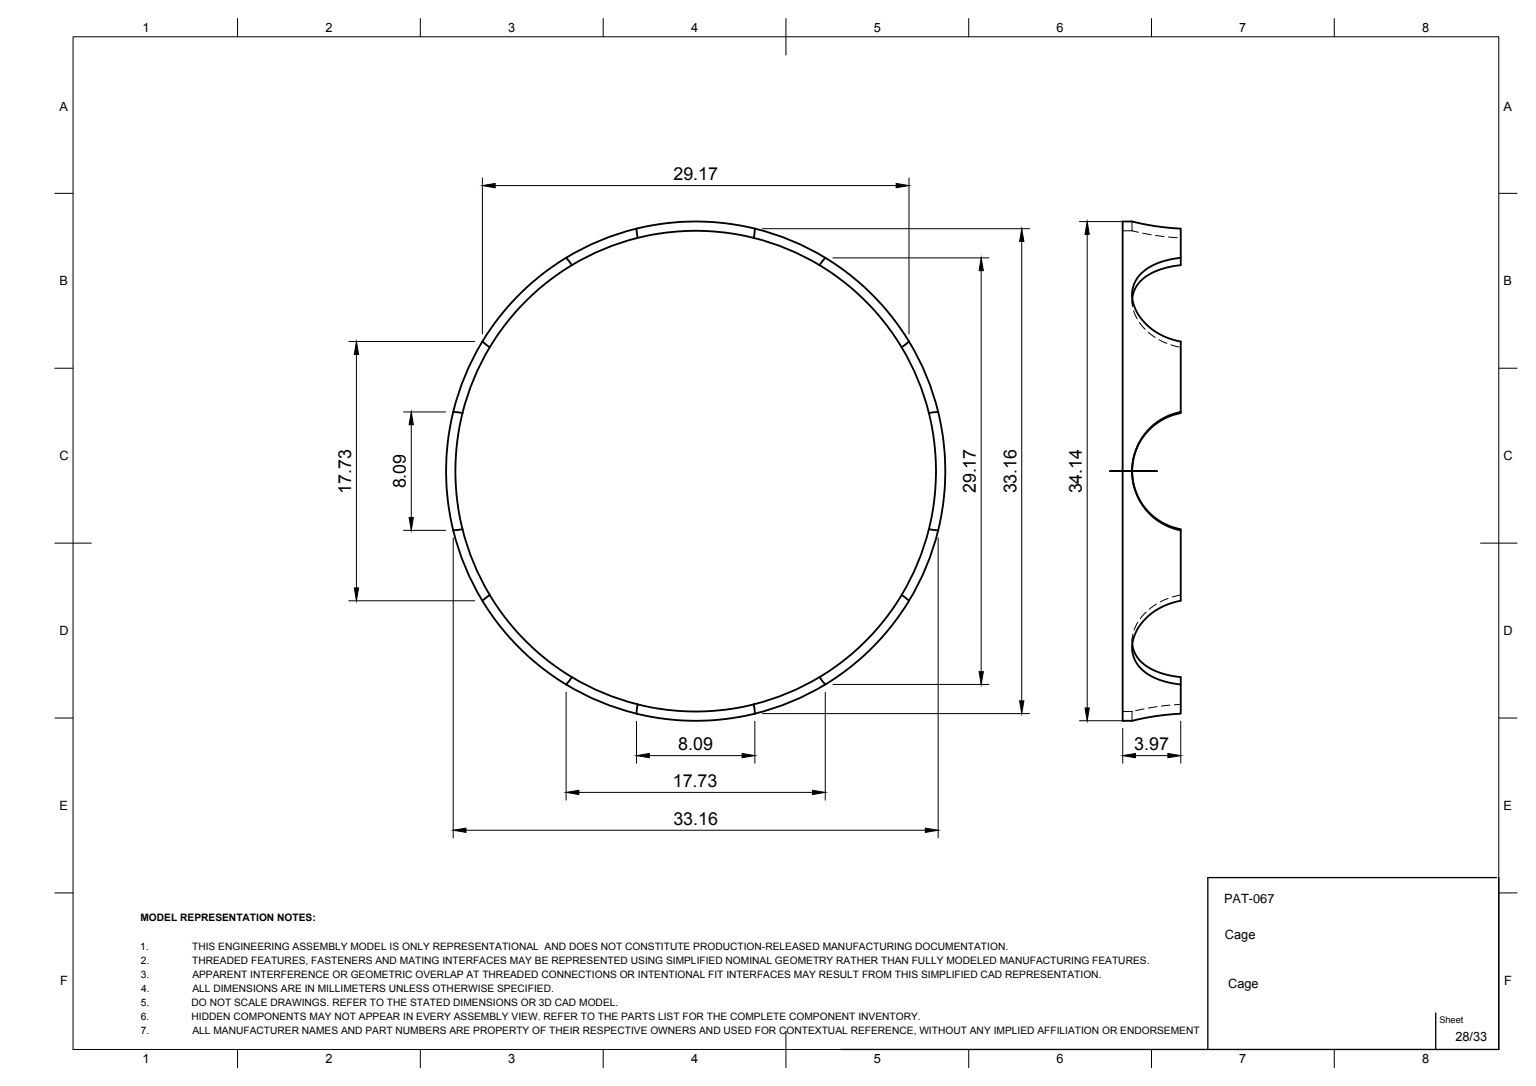
ISO-10303-21;
HEADER;
/* Generated by software containing ST-Developer
 * from STEP Tools, Inc. (www.steptools.com) 
 */

FILE_DESCRIPTION(
/* description */ ('Lifting hook block with sheave'),
/* implementation_level */ '2;1');

FILE_NAME(
/* name */ 'Cage.step',
/* time_stamp */ '2026-10-28T03:23:54-07:00',
/* author */ (''),
/* organization */ (''),
/* preprocessor_version */ 'ST-DEVELOPER v20.2',
/* originating_system */ 'Autodesk Translation Framework v15.17.0.0',
/* authorisation */ '');

FILE_SCHEMA (('AUTOMOTIVE_DESIGN { 1 0 10303 214 3 1 1 }'));
ENDSEC;

DATA;
#10=MECHANICAL_DESIGN_GEOMETRIC_PRESENTATION_REPRESENTATION('',(#381),#9391);
#11=B_SPLINE_CURVE_WITH_KNOTS('',3,(#8590,#8591,#8592,#8593,#8594,#8595,
#8596,#8597,#8598,#8599,#8600,#8601,#8602,#8603,#8604,#8605,#8606,#8607,
#8608,#8609,#8610,#8611),.UNSPECIFIED.,.F.,.F.,(4,2,2,2,2,2,2,2,2,2,4),
(0.0789094028588958,0.210573405340968,0.315860108011452,0.421146810681936,
0.522142632548711,0.623138454415485,0.72413427628226,0.825130098149035,
0.930416800819519,1.03570350349,1.16736750597208),.UNSPECIFIED.);
#12=B_SPLINE_CURVE_WITH_KNOTS('',3,(#8615,#8616,#8617,#8618,#8619,#8620,
#8621,#8622,#8623,#8624,#8625,#8626,#8627,#8628,#8629,#8630,#8631,#8632,
#8633,#8634,#8635,#8636),.UNSPECIFIED.,.F.,.F.,(4,2,2,2,2,2,2,2,2,2,4),
(0.0774793363974613,0.142088896491891,0.284177792983782,0.411119756996526,
0.514392970548519,0.617666184100513,0.720939397652506,0.8242126112045,0.951154575217244,
1.09324347170913,1.15785303180356),.UNSPECIFIED.);
#13=B_SPLINE_CURVE_WITH_KNOTS('',3,(#8642,#8643,#8644,#8645,#8646,#8647,
#8648,#8649,#8650,#8651,#8652,#8653,#8654,#8655,#8656,#8657,#8658,#8659,
#8660,#8661,#8662,#8663),.UNSPECIFIED.,.F.,.F.,(4,2,2,2,2,2,2,2,2,2,4),
(0.0774793363974613,0.142088896491891,0.284177792983782,0.411119756996525,
0.514392970548519,0.617666184100513,0.720939397652506,0.8242126112045,0.951154575217243,
1.09324347170913,1.15785303180356),.UNSPECIFIED.);
#14=B_SPLINE_CURVE_WITH_KNOTS('',3,(#8667,#8668,#8669,#8670,#8671,#8672,
#8673,#8674,#8675,#8676,#8677,#8678,#8679,#8680,#8681,#8682,#8683,#8684,
#8685,#8686,#8687,#8688),.UNSPECIFIED.,.F.,.F.,(4,2,2,2,2,2,2,2,2,2,4),
(0.0774793363974614,0.142088896491891,0.284177792983781,0.411119756996525,
0.514392970548519,0.617666184100512,0.720939397652506,0.824212611204499,
0.951154575217243,1.09324347170913,1.15785303180356),.UNSPECIFIED.);
#15=B_SPLINE_CURVE_WITH_KNOTS('',3,(#8692,#8693,#8694,#8695,#8696,#8697,
#8698,#8699,#8700,#8701,#8702,#8703),.UNSPECIFIED.,.F.,.F.,(4,2,2,2,2,4),
(0.0774793363974613,0.142088896491891,0.284177792983781,0.411119756996525,
0.514392970548519,0.617666184100512),.UNSPECIFIED.);
#16=B_SPLINE_CURVE_WITH_KNOTS('',3,(#8708,#8709,#8710,#8711,#8712,#8713,
#8714,#8715,#8716,#8717,#8718,#8719),.UNSPECIFIED.,.F.,.F.,(4,2,2,2,2,4),
(0.617666184100512,0.720939397652506,0.824212611204499,0.951154575217243,
1.09324347170913,1.15785303180356),.UNSPECIFIED.);
#17=B_SPLINE_CURVE_WITH_KNOTS('',3,(#8723,#8724,#8725,#8726,#8727,#8728,
#8729,#8730,#8731,#8732,#8733,#8734,#8735,#8736,#8737,#8738,#8739,#8740,
#8741,#8742,#8743,#8744),.UNSPECIFIED.,.F.,.F.,(4,2,2,2,2,2,2,2,2,2,4),
(0.0774793363974613,0.142088896491891,0.284177792983782,0.411119756996526,
0.514392970548519,0.617666184100513,0.720939397652507,0.8242126112045,0.951154575217245,
1.09324347170914,1.15785303180356),.UNSPECIFIED.);
#18=B_SPLINE_CURVE_WITH_KNOTS('',3,(#8748,#8749,#8750,#8751,#8752,#8753,
#8754,#8755,#8756,#8757,#8758,#8759,#8760,#8761,#8762,#8763,#8764,#8765,
#8766,#8767,#8768,#8769),.UNSPECIFIED.,.F.,.F.,(4,2,2,2,2,2,2,2,2,2,4),
(0.0774793363974613,0.142088896491891,0.284177792983782,0.411119756996526,
0.514392970548519,0.617666184100513,0.720939397652506,0.824212611204499,
0.951154575217243,1.09324347170913,1.15785303180356),.UNSPECIFIED.);
#19=B_SPLINE_CURVE_WITH_KNOTS('',3,(#8773,#8774,#8775,#8776,#8777,#8778,
#8779,#8780,#8781,#8782,#8783,#8784,#8785,#8786,#8787,#8788,#8789,#8790,
#8791,#8792,#8793,#8794),.UNSPECIFIED.,.F.,.F.,(4,2,2,2,2,2,2,2,2,2,4),
(0.0774793363974613,0.142088896491891,0.284177792983782,0.411119756996526,
0.514392970548519,0.617666184100513,0.720939397652506,0.8242126112045,0.951154575217244,
1.09324347170913,1.15785303180356),.UNSPECIFIED.);
#20=B_SPLINE_CURVE_WITH_KNOTS('',3,(#8798,#8799,#8800,#8801,#8802,#8803,
#8804,#8805,#8806,#8807,#8808,#8809,#8810,#8811,#8812,#8813,#8814,#8815,
#8816,#8817,#8818,#8819),.UNSPECIFIED.,.F.,.F.,(4,2,2,2,2,2,2,2,2,2,4),
(0.0774793363974613,0.142088896491891,0.284177792983782,0.411119756996526,
0.514392970548519,0.617666184100513,0.720939397652506,0.8242126112045,0.951154575217243,
1.09324347170913,1.15785303180356),.UNSPECIFIED.);
#21=B_SPLINE_CURVE_WITH_KNOTS('',3,(#8827,#8828,#8829,#8830,#8831,#8832,
#8833,#8834,#8835,#8836,#8837,#8838,#8839,#8840,#8841,#8842,#8843,#8844,
#8845,#8846,#8847,#8848),.UNSPECIFIED.,.F.,.F.,(4,2,2,2,2,2,2,2,2,2,4),
(0.0789094028588958,0.210573405340968,0.315860108011452,0.421146810681936,
0.522142632548711,0.623138454415485,0.72413427628226,0.825130098149035,
0.930416800819519,1.03570350349,1.16736750597208),.UNSPECIFIED.);
#22=B_SPLINE_CURVE_WITH_KNOTS('',3,(#8856,#8857,#8858,#8859,#8860,#8861,
#8862,#8863,#8864,#8865,#8866,#8867,#8868,#8869,#8870,#8871,#8872,#8873,
#8874,#8875,#8876,#8877),.UNSPECIFIED.,.F.,.F.,(4,2,2,2,2,2,2,2,2,2,4),
(0.0789094028588958,0.210573405340969,0.315860108011453,0.421146810681937,
0.522142632548712,0.623138454415486,0.724134276282261,0.825130098149035,
0.930416800819519,1.03570350349,1.16736750597208),.UNSPECIFIED.);
#23=B_SPLINE_CURVE_WITH_KNOTS('',3,(#8886,#8887,#8888,#8889,#8890,#8891,
#8892,#8893,#8894,#8895,#8896,#8897),.UNSPECIFIED.,.F.,.F.,(4,2,2,2,2,4),
(0.0789094028588958,0.210573405340968,0.315860108011452,0.421146810681937,
0.522142632548711,0.623138454415486),.UNSPECIFIED.);
#24=B_SPLINE_CURVE_WITH_KNOTS('',3,(#8899,#8900,#8901,#8902,#8903,#8904,
#8905,#8906,#8907,#8908,#8909,#8910),.UNSPECIFIED.,.F.,.F.,(4,2,2,2,2,4),
(0.623138454415486,0.72413427628226,0.825130098149035,0.930416800819519,
1.03570350349,1.16736750597208),.UNSPECIFIED.);
#25=B_SPLINE_CURVE_WITH_KNOTS('',3,(#8917,#8918,#8919,#8920,#8921,#8922,
#8923,#8924,#8925,#8926,#8927,#8928,#8929,#8930,#8931,#8932,#8933,#8934,
#8935,#8936,#8937,#8938),.UNSPECIFIED.,.F.,.F.,(4,2,2,2,2,2,2,2,2,2,4),
(0.0789094028588958,0.210573405340968,0.315860108011452,0.421146810681936,
0.522142632548711,0.623138454415486,0.72413427628226,0.825130098149035,
0.930416800819519,1.03570350349,1.16736750597208),.UNSPECIFIED.);
#26=B_SPLINE_CURVE_WITH_KNOTS('',3,(#8946,#8947,#8948,#8949,#8950,#8951,
#8952,#8953,#8954,#8955,#8956,#8957,#8958,#8959,#8960,#8961,#8962,#8963,
#8964,#8965,#8966,#8967),.UNSPECIFIED.,.F.,.F.,(4,2,2,2,2,2,2,2,2,2,4),
(0.0789094028588957,0.210573405340968,0.315860108011452,0.421146810681936,
0.522142632548711,0.623138454415485,0.72413427628226,0.825130098149035,
0.930416800819519,1.03570350349,1.16736750597207),.UNSPECIFIED.);
#27=B_SPLINE_CURVE_WITH_KNOTS('',3,(#8975,#8976,#8977,#8978,#8979,#8980,
#8981,#8982,#8983,#8984,#8985,#8986,#8987,#8988,#8989,#8990,#8991,#8992,
#8993,#8994,#8995,#8996),.UNSPECIFIED.,.F.,.F.,(4,2,2,2,2,2,2,2,2,2,4),
(0.0789094028588958,0.210573405340968,0.315860108011452,0.421146810681936,
0.522142632548711,0.623138454415486,0.72413427628226,0.825130098149035,
0.930416800819519,1.03570350349,1.16736750597208),.UNSPECIFIED.);
#28=B_SPLINE_CURVE_WITH_KNOTS('',3,(#9005,#9006,#9007,#9008,#9009,#9010,
#9011,#9012,#9013,#9014,#9015,#9016,#9017,#9018,#9019,#9020,#9021,#9022,
#9023,#9024,#9025,#9026),.UNSPECIFIED.,.F.,.F.,(4,2,2,2,2,2,2,2,2,2,4),
(0.0789094028588958,0.210573405340968,0.315860108011452,0.421146810681936,
0.522142632548711,0.623138454415485,0.72413427628226,0.825130098149035,
0.930416800819519,1.03570350349,1.16736750597208),.UNSPECIFIED.);
#37=SPHERICAL_SURFACE('',#5741,0.412776);
#38=SPHERICAL_SURFACE('',#5757,0.412776);
#39=SPHERICAL_SURFACE('',#5762,0.412776);
#40=SPHERICAL_SURFACE('',#5767,0.412776);
#41=SPHERICAL_SURFACE('',#5772,0.412776);
#42=SPHERICAL_SURFACE('',#5777,0.412776);
#43=SPHERICAL_SURFACE('',#5782,0.412776);
#44=SPHERICAL_SURFACE('',#5790,0.412776);
#314=SHAPE_REPRESENTATION_RELATIONSHIP('SRR','None',#9547,#344);
#344=ADVANCED_BREP_SHAPE_REPRESENTATION('',(#417),#9382);
#381=STYLED_ITEM('',(#9759),#417);
#417=MANIFOLD_SOLID_BREP('Continuous crown cage',#4919);
#636=LINE('',#8705,#924);
#637=LINE('',#9001,#925);
#924=VECTOR('',#7119,1.706752);
#925=VECTOR('',#7196,1.643248);
#1087=CYLINDRICAL_SURFACE('',#5744,1.706752);
#1088=CYLINDRICAL_SURFACE('',#5784,1.643248);
#1206=FACE_BOUND('',#1839,.T.);
#1433=FACE_OUTER_BOUND('',#1821,.T.);
#1434=FACE_OUTER_BOUND('',#1822,.T.);
#1435=FACE_OUTER_BOUND('',#1823,.T.);
#1436=FACE_OUTER_BOUND('',#1824,.T.);
#1437=FACE_OUTER_BOUND('',#1825,.T.);
#1438=FACE_OUTER_BOUND('',#1826,.T.);
#1439=FACE_OUTER_BOUND('',#1827,.T.);
#1440=FACE_OUTER_BOUND('',#1828,.T.);
#1441=FACE_OUTER_BOUND('',#1829,.T.);
#1442=FACE_OUTER_BOUND('',#1830,.T.);
#1443=FACE_OUTER_BOUND('',#1831,.T.);
#1444=FACE_OUTER_BOUND('',#1832,.T.);
#1445=FACE_OUTER_BOUND('',#1833,.T.);
#1446=FACE_OUTER_BOUND('',#1834,.T.);
#1447=FACE_OUTER_BOUND('',#1835,.T.);
#1448=FACE_OUTER_BOUND('',#1836,.T.);
#1449=FACE_OUTER_BOUND('',#1837,.T.);
#1450=FACE_OUTER_BOUND('',#1838,.T.);
#1451=FACE_OUTER_BOUND('',#1840,.T.);
#1821=EDGE_LOOP('',(#4114,#4115,#4116,#4117));
#1822=EDGE_LOOP('',(#4118,#4119,#4120,#4121,#4122,#4123,#4124,#4125,#4126,
#4127,#4128,#4129,#4130,#4131,#4132,#4133,#4134,#4135,#4136,#4137));
#1823=EDGE_LOOP('',(#4138,#4139,#4140,#4141));
#1824=EDGE_LOOP('',(#4142,#4143,#4144,#4145));
#1825=EDGE_LOOP('',(#4146,#4147,#4148,#4149));
#1826=EDGE_LOOP('',(#4150,#4151,#4152,#4153));
#1827=EDGE_LOOP('',(#4154,#4155,#4156,#4157));
#1828=EDGE_LOOP('',(#4158,#4159,#4160,#4161,#4162,#4163));
#1829=EDGE_LOOP('',(#4164,#4165,#4166,#4167));
#1830=EDGE_LOOP('',(#4168,#4169,#4170,#4171));
#1831=EDGE_LOOP('',(#4172,#4173,#4174,#4175));
#1832=EDGE_LOOP('',(#4176,#4177,#4178,#4179));
#1833=EDGE_LOOP('',(#4180,#4181,#4182,#4183));
#1834=EDGE_LOOP('',(#4184,#4185,#4186,#4187));
#1835=EDGE_LOOP('',(#4188,#4189,#4190,#4191,#4192,#4193,#4194,#4195,#4196,
#4197,#4198,#4199,#4200,#4201,#4202,#4203,#4204,#4205,#4206,#4207));
#1836=EDGE_LOOP('',(#4208,#4209,#4210,#4211));
#1837=EDGE_LOOP('',(#4212,#4213,#4214,#4215));
#1838=EDGE_LOOP('',(#4216));
#1839=EDGE_LOOP('',(#4217));
#1840=EDGE_LOOP('',(#4218,#4219,#4220,#4221));
#2133=CIRCLE('',#5742,0.405071403305639);
#2134=CIRCLE('',#5743,0.405071403305639);
#2135=CIRCLE('',#5745,1.706752);
#2136=CIRCLE('',#5746,1.706752);
#2137=CIRCLE('',#5747,1.706752);
#2138=CIRCLE('',#5748,1.706752);
#2139=CIRCLE('',#5749,1.706752);
#2140=CIRCLE('',#5750,1.706752);
#2141=CIRCLE('',#5751,1.706752);
#2142=CIRCLE('',#5752,1.706752);
#2143=CIRCLE('',#5753,1.706752);
#2144=CIRCLE('',#5755,1.643248);
#2145=CIRCLE('',#5756,0.405071403305639);
#2146=CIRCLE('',#5758,0.405071403305639);
#2147=CIRCLE('',#5760,1.643248);
#2148=CIRCLE('',#5761,0.405071403305639);
#2149=CIRCLE('',#5763,0.405071403305639);
#2150=CIRCLE('',#5765,1.643248);
#2151=CIRCLE('',#5766,0.405071403305639);
#2152=CIRCLE('',#5768,0.405071403305639);
#2153=CIRCLE('',#5770,1.643248);
#2154=CIRCLE('',#5771,0.405071403305639);
#2155=CIRCLE('',#5773,0.405071403305639);
#2156=CIRCLE('',#5775,1.643248);
#2157=CIRCLE('',#5776,0.405071403305639);
#2158=CIRCLE('',#5778,0.405071403305639);
#2159=CIRCLE('',#5780,1.643248);
#2160=CIRCLE('',#5781,0.405071403305639);
#2161=CIRCLE('',#5783,0.405071403305639);
#2162=CIRCLE('',#5785,1.643248);
#2163=CIRCLE('',#5786,1.643248);
#2164=CIRCLE('',#5787,1.643248);
#2165=CIRCLE('',#5789,0.405071403305639);
#2166=CIRCLE('',#5791,0.405071403305639);
#2508=VERTEX_POINT('',#8588);
#2509=VERTEX_POINT('',#8589);
#2510=VERTEX_POINT('',#8612);
#2511=VERTEX_POINT('',#8614);
#2512=VERTEX_POINT('',#8639);
#2513=VERTEX_POINT('',#8641);
#2514=VERTEX_POINT('',#8664);
#2515=VERTEX_POINT('',#8666);
#2516=VERTEX_POINT('',#8689);
#2517=VERTEX_POINT('',#8691);
#2518=VERTEX_POINT('',#8704);
#2519=VERTEX_POINT('',#8707);
#2520=VERTEX_POINT('',#8720);
#2521=VERTEX_POINT('',#8722);
#2522=VERTEX_POINT('',#8745);
#2523=VERTEX_POINT('',#8747);
#2524=VERTEX_POINT('',#8770);
#2525=VERTEX_POINT('',#8772);
#2526=VERTEX_POINT('',#8795);
#2527=VERTEX_POINT('',#8797);
#2528=VERTEX_POINT('',#8822);
#2529=VERTEX_POINT('',#8826);
#2530=VERTEX_POINT('',#8851);
#2531=VERTEX_POINT('',#8855);
#2532=VERTEX_POINT('',#8880);
#2533=VERTEX_POINT('',#8884);
#2534=VERTEX_POINT('',#8885);
#2535=VERTEX_POINT('',#8912);
#2536=VERTEX_POINT('',#8916);
#2537=VERTEX_POINT('',#8941);
#2538=VERTEX_POINT('',#8945);
#2539=VERTEX_POINT('',#8970);
#2540=VERTEX_POINT('',#8974);
#2541=VERTEX_POINT('',#8999);
#2542=VERTEX_POINT('',#9002);
#2543=VERTEX_POINT('',#9004);
#3061=EDGE_CURVE('',#2508,#2509,#11,.T.);
#3062=EDGE_CURVE('',#2510,#2508,#2133,.T.);
#3063=EDGE_CURVE('',#2511,#2510,#12,.T.);
#3064=EDGE_CURVE('',#2509,#2511,#2134,.T.);
#3065=EDGE_CURVE('',#2512,#2510,#2135,.T.);
#3066=EDGE_CURVE('',#2512,#2513,#13,.T.);
#3067=EDGE_CURVE('',#2514,#2513,#2136,.T.);
#3068=EDGE_CURVE('',#2514,#2515,#14,.T.);
#3069=EDGE_CURVE('',#2516,#2515,#2137,.T.);
#3070=EDGE_CURVE('',#2516,#2517,#15,.T.);
#3071=EDGE_CURVE('',#2517,#2518,#636,.T.);
#3072=EDGE_CURVE('',#2518,#2518,#2138,.T.);
#3073=EDGE_CURVE('',#2517,#2519,#16,.T.);
#3074=EDGE_CURVE('',#2520,#2519,#2139,.T.);
#3075=EDGE_CURVE('',#2520,#2521,#17,.T.);
#3076=EDGE_CURVE('',#2522,#2521,#2140,.T.);
#3077=EDGE_CURVE('',#2522,#2523,#18,.T.);
#3078=EDGE_CURVE('',#2524,#2523,#2141,.T.);
#3079=EDGE_CURVE('',#2524,#2525,#19,.T.);
#3080=EDGE_CURVE('',#2526,#2525,#2142,.T.);
#3081=EDGE_CURVE('',#2526,#2527,#20,.T.);
#3082=EDGE_CURVE('',#2511,#2527,#2143,.T.);
#3083=EDGE_CURVE('',#2508,#2528,#2144,.T.);
#3084=EDGE_CURVE('',#2528,#2512,#2145,.T.);
#3085=EDGE_CURVE('',#2529,#2528,#21,.T.);
#3086=EDGE_CURVE('',#2513,#2529,#2146,.T.);
#3087=EDGE_CURVE('',#2529,#2530,#2147,.T.);
#3088=EDGE_CURVE('',#2530,#2514,#2148,.T.);
#3089=EDGE_CURVE('',#2531,#2530,#22,.T.);
#3090=EDGE_CURVE('',#2515,#2531,#2149,.T.);
#3091=EDGE_CURVE('',#2531,#2532,#2150,.T.);
#3092=EDGE_CURVE('',#2532,#2516,#2151,.T.);
#3093=EDGE_CURVE('',#2533,#2534,#23,.T.);
#3094=EDGE_CURVE('',#2519,#2533,#2152,.T.);
#3095=EDGE_CURVE('',#2534,#2532,#24,.T.);
#3096=EDGE_CURVE('',#2533,#2535,#2153,.T.);
#3097=EDGE_CURVE('',#2535,#2520,#2154,.T.);
#3098=EDGE_CURVE('',#2536,#2535,#25,.T.);
#3099=EDGE_CURVE('',#2521,#2536,#2155,.T.);
#3100=EDGE_CURVE('',#2536,#2537,#2156,.T.);
#3101=EDGE_CURVE('',#2537,#2522,#2157,.T.);
#3102=EDGE_CURVE('',#2538,#2537,#26,.T.);
#3103=EDGE_CURVE('',#2523,#2538,#2158,.T.);
#3104=EDGE_CURVE('',#2538,#2539,#2159,.T.);
#3105=EDGE_CURVE('',#2539,#2524,#2160,.T.);
#3106=EDGE_CURVE('',#2540,#2539,#27,.T.);
#3107=EDGE_CURVE('',#2525,#2540,#2161,.T.);
#3108=EDGE_CURVE('',#2541,#2541,#2162,.T.);
#3109=EDGE_CURVE('',#2541,#2534,#637,.T.);
#3110=EDGE_CURVE('',#2542,#2509,#2163,.T.);
#3111=EDGE_CURVE('',#2542,#2543,#28,.T.);
#3112=EDGE_CURVE('',#2540,#2543,#2164,.T.);
#3113=EDGE_CURVE('',#2527,#2542,#2165,.T.);
#3114=EDGE_CURVE('',#2543,#2526,#2166,.T.);
#4114=ORIENTED_EDGE('',*,*,#3061,.F.);
#4115=ORIENTED_EDGE('',*,*,#3062,.F.);
#4116=ORIENTED_EDGE('',*,*,#3063,.F.);
#4117=ORIENTED_EDGE('',*,*,#3064,.F.);
#4118=ORIENTED_EDGE('',*,*,#3063,.T.);
#4119=ORIENTED_EDGE('',*,*,#3065,.F.);
#4120=ORIENTED_EDGE('',*,*,#3066,.T.);
#4121=ORIENTED_EDGE('',*,*,#3067,.F.);
#4122=ORIENTED_EDGE('',*,*,#3068,.T.);
#4123=ORIENTED_EDGE('',*,*,#3069,.F.);
#4124=ORIENTED_EDGE('',*,*,#3070,.T.);
#4125=ORIENTED_EDGE('',*,*,#3071,.T.);
#4126=ORIENTED_EDGE('',*,*,#3072,.F.);
#4127=ORIENTED_EDGE('',*,*,#3071,.F.);
#4128=ORIENTED_EDGE('',*,*,#3073,.T.);
#4129=ORIENTED_EDGE('',*,*,#3074,.F.);
#4130=ORIENTED_EDGE('',*,*,#3075,.T.);
#4131=ORIENTED_EDGE('',*,*,#3076,.F.);
#4132=ORIENTED_EDGE('',*,*,#3077,.T.);
#4133=ORIENTED_EDGE('',*,*,#3078,.F.);
#4134=ORIENTED_EDGE('',*,*,#3079,.T.);
#4135=ORIENTED_EDGE('',*,*,#3080,.F.);
#4136=ORIENTED_EDGE('',*,*,#3081,.T.);
#4137=ORIENTED_EDGE('',*,*,#3082,.F.);
#4138=ORIENTED_EDGE('',*,*,#3062,.T.);
#4139=ORIENTED_EDGE('',*,*,#3083,.T.);
#4140=ORIENTED_EDGE('',*,*,#3084,.T.);
#4141=ORIENTED_EDGE('',*,*,#3065,.T.);
#4142=ORIENTED_EDGE('',*,*,#3085,.F.);
#4143=ORIENTED_EDGE('',*,*,#3086,.F.);
#4144=ORIENTED_EDGE('',*,*,#3066,.F.);
#4145=ORIENTED_EDGE('',*,*,#3084,.F.);
#4146=ORIENTED_EDGE('',*,*,#3086,.T.);
#4147=ORIENTED_EDGE('',*,*,#3087,.T.);
#4148=ORIENTED_EDGE('',*,*,#3088,.T.);
#4149=ORIENTED_EDGE('',*,*,#3067,.T.);
#4150=ORIENTED_EDGE('',*,*,#3089,.F.);
#4151=ORIENTED_EDGE('',*,*,#3090,.F.);
#4152=ORIENTED_EDGE('',*,*,#3068,.F.);
#4153=ORIENTED_EDGE('',*,*,#3088,.F.);
#4154=ORIENTED_EDGE('',*,*,#3090,.T.);
#4155=ORIENTED_EDGE('',*,*,#3091,.T.);
#4156=ORIENTED_EDGE('',*,*,#3092,.T.);
#4157=ORIENTED_EDGE('',*,*,#3069,.T.);
#4158=ORIENTED_EDGE('',*,*,#3093,.F.);
#4159=ORIENTED_EDGE('',*,*,#3094,.F.);
#4160=ORIENTED_EDGE('',*,*,#3073,.F.);
#4161=ORIENTED_EDGE('',*,*,#3070,.F.);
#4162=ORIENTED_EDGE('',*,*,#3092,.F.);
#4163=ORIENTED_EDGE('',*,*,#3095,.F.);
#4164=ORIENTED_EDGE('',*,*,#3094,.T.);
#4165=ORIENTED_EDGE('',*,*,#3096,.T.);
#4166=ORIENTED_EDGE('',*,*,#3097,.T.);
#4167=ORIENTED_EDGE('',*,*,#3074,.T.);
#4168=ORIENTED_EDGE('',*,*,#3098,.F.);
#4169=ORIENTED_EDGE('',*,*,#3099,.F.);
#4170=ORIENTED_EDGE('',*,*,#3075,.F.);
#4171=ORIENTED_EDGE('',*,*,#3097,.F.);
#4172=ORIENTED_EDGE('',*,*,#3099,.T.);
#4173=ORIENTED_EDGE('',*,*,#3100,.T.);
#4174=ORIENTED_EDGE('',*,*,#3101,.T.);
#4175=ORIENTED_EDGE('',*,*,#3076,.T.);
#4176=ORIENTED_EDGE('',*,*,#3102,.F.);
#4177=ORIENTED_EDGE('',*,*,#3103,.F.);
#4178=ORIENTED_EDGE('',*,*,#3077,.F.);
#4179=ORIENTED_EDGE('',*,*,#3101,.F.);
#4180=ORIENTED_EDGE('',*,*,#3103,.T.);
#4181=ORIENTED_EDGE('',*,*,#3104,.T.);
#4182=ORIENTED_EDGE('',*,*,#3105,.T.);
#4183=ORIENTED_EDGE('',*,*,#3078,.T.);
#4184=ORIENTED_EDGE('',*,*,#3079,.F.);
#4185=ORIENTED_EDGE('',*,*,#3105,.F.);
#4186=ORIENTED_EDGE('',*,*,#3106,.F.);
#4187=ORIENTED_EDGE('',*,*,#3107,.F.);
#4188=ORIENTED_EDGE('',*,*,#3108,.F.);
#4189=ORIENTED_EDGE('',*,*,#3109,.T.);
#4190=ORIENTED_EDGE('',*,*,#3095,.T.);
#4191=ORIENTED_EDGE('',*,*,#3091,.F.);
#4192=ORIENTED_EDGE('',*,*,#3089,.T.);
#4193=ORIENTED_EDGE('',*,*,#3087,.F.);
#4194=ORIENTED_EDGE('',*,*,#3085,.T.);
#4195=ORIENTED_EDGE('',*,*,#3083,.F.);
#4196=ORIENTED_EDGE('',*,*,#3061,.T.);
#4197=ORIENTED_EDGE('',*,*,#3110,.F.);
#4198=ORIENTED_EDGE('',*,*,#3111,.T.);
#4199=ORIENTED_EDGE('',*,*,#3112,.F.);
#4200=ORIENTED_EDGE('',*,*,#3106,.T.);
#4201=ORIENTED_EDGE('',*,*,#3104,.F.);
#4202=ORIENTED_EDGE('',*,*,#3102,.T.);
#4203=ORIENTED_EDGE('',*,*,#3100,.F.);
#4204=ORIENTED_EDGE('',*,*,#3098,.T.);
#4205=ORIENTED_EDGE('',*,*,#3096,.F.);
#4206=ORIENTED_EDGE('',*,*,#3093,.T.);
#4207=ORIENTED_EDGE('',*,*,#3109,.F.);
#4208=ORIENTED_EDGE('',*,*,#3064,.T.);
#4209=ORIENTED_EDGE('',*,*,#3082,.T.);
#4210=ORIENTED_EDGE('',*,*,#3113,.T.);
#4211=ORIENTED_EDGE('',*,*,#3110,.T.);
#4212=ORIENTED_EDGE('',*,*,#3081,.F.);
#4213=ORIENTED_EDGE('',*,*,#3114,.F.);
#4214=ORIENTED_EDGE('',*,*,#3111,.F.);
#4215=ORIENTED_EDGE('',*,*,#3113,.F.);
#4216=ORIENTED_EDGE('',*,*,#3072,.T.);
#4217=ORIENTED_EDGE('',*,*,#3108,.T.);
#4218=ORIENTED_EDGE('',*,*,#3107,.T.);
#4219=ORIENTED_EDGE('',*,*,#3112,.T.);
#4220=ORIENTED_EDGE('',*,*,#3114,.T.);
#4221=ORIENTED_EDGE('',*,*,#3080,.T.);
#4551=PLANE('',#5754);
#4552=PLANE('',#5759);
#4553=PLANE('',#5764);
#4554=PLANE('',#5769);
#4555=PLANE('',#5774);
#4556=PLANE('',#5779);
#4557=PLANE('',#5788);
#4558=PLANE('',#5792);
#4559=PLANE('',#5793);
#4809=ADVANCED_FACE('',(#1433),#37,.F.);
#4810=ADVANCED_FACE('',(#1434),#1087,.T.);
#4811=ADVANCED_FACE('',(#1435),#4551,.T.);
#4812=ADVANCED_FACE('',(#1436),#38,.F.);
#4813=ADVANCED_FACE('',(#1437),#4552,.T.);
#4814=ADVANCED_FACE('',(#1438),#39,.F.);
#4815=ADVANCED_FACE('',(#1439),#4553,.T.);
#4816=ADVANCED_FACE('',(#1440),#40,.F.);
#4817=ADVANCED_FACE('',(#1441),#4554,.T.);
#4818=ADVANCED_FACE('',(#1442),#41,.F.);
#4819=ADVANCED_FACE('',(#1443),#4555,.T.);
#4820=ADVANCED_FACE('',(#1444),#42,.F.);
#4821=ADVANCED_FACE('',(#1445),#4556,.T.);
#4822=ADVANCED_FACE('',(#1446),#43,.F.);
#4823=ADVANCED_FACE('',(#1447),#1088,.F.);
#4824=ADVANCED_FACE('',(#1448),#4557,.T.);
#4825=ADVANCED_FACE('',(#1449),#44,.F.);
#4826=ADVANCED_FACE('',(#1450,#1206),#4558,.T.);
#4827=ADVANCED_FACE('',(#1451),#4559,.T.);
#4919=CLOSED_SHELL('',(#4809,#4810,#4811,#4812,#4813,#4814,#4815,#4816,
#4817,#4818,#4819,#4820,#4821,#4822,#4823,#4824,#4825,#4826,#4827));
#5740=AXIS2_PLACEMENT_3D('',#8586,#7103,#7104);
#5741=AXIS2_PLACEMENT_3D('',#8587,#7105,#7106);
#5742=AXIS2_PLACEMENT_3D('',#8613,#7107,#7108);
#5743=AXIS2_PLACEMENT_3D('',#8637,#7109,#7110);
#5744=AXIS2_PLACEMENT_3D('',#8638,#7111,#7112);
#5745=AXIS2_PLACEMENT_3D('',#8640,#7113,#7114);
#5746=AXIS2_PLACEMENT_3D('',#8665,#7115,#7116);
#5747=AXIS2_PLACEMENT_3D('',#8690,#7117,#7118);
#5748=AXIS2_PLACEMENT_3D('',#8706,#7120,#7121);
#5749=AXIS2_PLACEMENT_3D('',#8721,#7122,#7123);
#5750=AXIS2_PLACEMENT_3D('',#8746,#7124,#7125);
#5751=AXIS2_PLACEMENT_3D('',#8771,#7126,#7127);
#5752=AXIS2_PLACEMENT_3D('',#8796,#7128,#7129);
#5753=AXIS2_PLACEMENT_3D('',#8820,#7130,#7131);
#5754=AXIS2_PLACEMENT_3D('',#8821,#7132,#7133);
#5755=AXIS2_PLACEMENT_3D('',#8823,#7134,#7135);
#5756=AXIS2_PLACEMENT_3D('',#8824,#7136,#7137);
#5757=AXIS2_PLACEMENT_3D('',#8825,#7138,#7139);
#5758=AXIS2_PLACEMENT_3D('',#8849,#7140,#7141);
#5759=AXIS2_PLACEMENT_3D('',#8850,#7142,#7143);
#5760=AXIS2_PLACEMENT_3D('',#8852,#7144,#7145);
#5761=AXIS2_PLACEMENT_3D('',#8853,#7146,#7147);
#5762=AXIS2_PLACEMENT_3D('',#8854,#7148,#7149);
#5763=AXIS2_PLACEMENT_3D('',#8878,#7150,#7151);
#5764=AXIS2_PLACEMENT_3D('',#8879,#7152,#7153);
#5765=AXIS2_PLACEMENT_3D('',#8881,#7154,#7155);
#5766=AXIS2_PLACEMENT_3D('',#8882,#7156,#7157);
#5767=AXIS2_PLACEMENT_3D('',#8883,#7158,#7159);
#5768=AXIS2_PLACEMENT_3D('',#8898,#7160,#7161);
#5769=AXIS2_PLACEMENT_3D('',#8911,#7162,#7163);
#5770=AXIS2_PLACEMENT_3D('',#8913,#7164,#7165);
#5771=AXIS2_PLACEMENT_3D('',#8914,#7166,#7167);
#5772=AXIS2_PLACEMENT_3D('',#8915,#7168,#7169);
#5773=AXIS2_PLACEMENT_3D('',#8939,#7170,#7171);
#5774=AXIS2_PLACEMENT_3D('',#8940,#7172,#7173);
#5775=AXIS2_PLACEMENT_3D('',#8942,#7174,#7175);
#5776=AXIS2_PLACEMENT_3D('',#8943,#7176,#7177);
#5777=AXIS2_PLACEMENT_3D('',#8944,#7178,#7179);
#5778=AXIS2_PLACEMENT_3D('',#8968,#7180,#7181);
#5779=AXIS2_PLACEMENT_3D('',#8969,#7182,#7183);
#5780=AXIS2_PLACEMENT_3D('',#8971,#7184,#7185);
#5781=AXIS2_PLACEMENT_3D('',#8972,#7186,#7187);
#5782=AXIS2_PLACEMENT_3D('',#8973,#7188,#7189);
#5783=AXIS2_PLACEMENT_3D('',#8997,#7190,#7191);
#5784=AXIS2_PLACEMENT_3D('',#8998,#7192,#7193);
#5785=AXIS2_PLACEMENT_3D('',#9000,#7194,#7195);
#5786=AXIS2_PLACEMENT_3D('',#9003,#7197,#7198);
#5787=AXIS2_PLACEMENT_3D('',#9027,#7199,#7200);
#5788=AXIS2_PLACEMENT_3D('',#9028,#7201,#7202);
#5789=AXIS2_PLACEMENT_3D('',#9029,#7203,#7204);
#5790=AXIS2_PLACEMENT_3D('',#9030,#7205,#7206);
#5791=AXIS2_PLACEMENT_3D('',#9031,#7207,#7208);
#5792=AXIS2_PLACEMENT_3D('',#9032,#7209,#7210);
#5793=AXIS2_PLACEMENT_3D('',#9033,#7211,#7212);
#7103=DIRECTION('axis',(0.,0.,1.));
#7104=DIRECTION('refdir',(1.,0.,0.));
#7105=DIRECTION('center_axis',(0.,0.,1.));
#7106=DIRECTION('ref_axis',(1.,0.,0.));
#7107=DIRECTION('center_axis',(0.,-1.,0.));
#7108=DIRECTION('ref_axis',(0.,0.,-1.));
#7109=DIRECTION('center_axis',(0.,-1.,0.));
#7110=DIRECTION('ref_axis',(0.,0.,-1.));
#7111=DIRECTION('center_axis',(0.,1.,0.));
#7112=DIRECTION('ref_axis',(1.,0.,0.));
#7113=DIRECTION('center_axis',(0.,1.,0.));
#7114=DIRECTION('ref_axis',(1.,0.,0.));
#7115=DIRECTION('center_axis',(0.,1.,0.));
#7116=DIRECTION('ref_axis',(1.,0.,0.));
#7117=DIRECTION('center_axis',(0.,1.,0.));
#7118=DIRECTION('ref_axis',(1.,0.,0.));
#7119=DIRECTION('',(0.,-1.,0.));
#7120=DIRECTION('center_axis',(0.,-1.,0.));
#7121=DIRECTION('ref_axis',(1.,0.,0.));
#7122=DIRECTION('center_axis',(0.,1.,0.));
#7123=DIRECTION('ref_axis',(1.,0.,0.));
#7124=DIRECTION('center_axis',(0.,1.,0.));
#7125=DIRECTION('ref_axis',(1.,0.,0.));
#7126=DIRECTION('center_axis',(0.,1.,0.));
#7127=DIRECTION('ref_axis',(1.,0.,0.));
#7128=DIRECTION('center_axis',(0.,1.,0.));
#7129=DIRECTION('ref_axis',(1.,0.,0.));
#7130=DIRECTION('center_axis',(0.,1.,0.));
#7131=DIRECTION('ref_axis',(1.,0.,0.));
#7132=DIRECTION('center_axis',(0.,1.,0.));
#7133=DIRECTION('ref_axis',(1.,0.,0.));
#7134=DIRECTION('center_axis',(0.,-1.,0.));
#7135=DIRECTION('ref_axis',(1.,0.,0.));
#7136=DIRECTION('center_axis',(0.,-1.,0.));
#7137=DIRECTION('ref_axis',(0.,0.,-1.));
#7138=DIRECTION('center_axis',(6.12323399573677E-17,0.,1.));
#7139=DIRECTION('ref_axis',(1.,0.,0.));
#7140=DIRECTION('center_axis',(0.,-1.,0.));
#7141=DIRECTION('ref_axis',(0.,0.,-1.));
#7142=DIRECTION('center_axis',(0.,1.,0.));
#7143=DIRECTION('ref_axis',(1.,0.,0.));
#7144=DIRECTION('center_axis',(0.,-1.,0.));
#7145=DIRECTION('ref_axis',(1.,0.,0.));
#7146=DIRECTION('center_axis',(0.,-1.,0.));
#7147=DIRECTION('ref_axis',(0.,0.,-1.));
#7148=DIRECTION('center_axis',(0.,0.,1.));
#7149=DIRECTION('ref_axis',(1.,0.,0.));
#7150=DIRECTION('center_axis',(0.,-1.,0.));
#7151=DIRECTION('ref_axis',(0.,0.,-1.));
#7152=DIRECTION('center_axis',(0.,1.,0.));
#7153=DIRECTION('ref_axis',(1.,0.,0.));
#7154=DIRECTION('center_axis',(0.,-1.,0.));
#7155=DIRECTION('ref_axis',(1.,0.,0.));
#7156=DIRECTION('center_axis',(0.,-1.,0.));
#7157=DIRECTION('ref_axis',(0.,0.,-1.));
#7158=DIRECTION('center_axis',(0.,0.,1.));
#7159=DIRECTION('ref_axis',(1.,0.,0.));
#7160=DIRECTION('center_axis',(0.,-1.,0.));
#7161=DIRECTION('ref_axis',(0.,0.,-1.));
#7162=DIRECTION('center_axis',(0.,1.,0.));
#7163=DIRECTION('ref_axis',(1.,0.,0.));
#7164=DIRECTION('center_axis',(0.,-1.,0.));
#7165=DIRECTION('ref_axis',(1.,0.,0.));
#7166=DIRECTION('center_axis',(0.,-1.,0.));
#7167=DIRECTION('ref_axis',(0.,0.,-1.));
#7168=DIRECTION('center_axis',(0.,0.,1.));
#7169=DIRECTION('ref_axis',(1.,0.,0.));
#7170=DIRECTION('center_axis',(0.,-1.,0.));
#7171=DIRECTION('ref_axis',(0.,0.,-1.));
#7172=DIRECTION('center_axis',(0.,1.,0.));
#7173=DIRECTION('ref_axis',(1.,0.,0.));
#7174=DIRECTION('center_axis',(0.,-1.,0.));
#7175=DIRECTION('ref_axis',(1.,0.,0.));
#7176=DIRECTION('center_axis',(0.,-1.,0.));
#7177=DIRECTION('ref_axis',(0.,0.,-1.));
#7178=DIRECTION('center_axis',(6.12323399573676E-17,0.,1.));
#7179=DIRECTION('ref_axis',(1.,0.,0.));
#7180=DIRECTION('center_axis',(0.,-1.,0.));
#7181=DIRECTION('ref_axis',(0.,0.,-1.));
#7182=DIRECTION('center_axis',(0.,1.,0.));
#7183=DIRECTION('ref_axis',(1.,0.,0.));
#7184=DIRECTION('center_axis',(0.,-1.,0.));
#7185=DIRECTION('ref_axis',(1.,0.,0.));
#7186=DIRECTION('center_axis',(0.,-1.,0.));
#7187=DIRECTION('ref_axis',(0.,0.,-1.));
#7188=DIRECTION('center_axis',(0.,0.,1.));
#7189=DIRECTION('ref_axis',(1.,0.,0.));
#7190=DIRECTION('center_axis',(0.,-1.,0.));
#7191=DIRECTION('ref_axis',(0.,0.,-1.));
#7192=DIRECTION('center_axis',(0.,1.,0.));
#7193=DIRECTION('ref_axis',(1.,0.,0.));
#7194=DIRECTION('center_axis',(0.,1.,0.));
#7195=DIRECTION('ref_axis',(1.,0.,0.));
#7196=DIRECTION('',(0.,1.,0.));
#7197=DIRECTION('center_axis',(0.,-1.,0.));
#7198=DIRECTION('ref_axis',(1.,0.,0.));
#7199=DIRECTION('center_axis',(0.,-1.,0.));
#7200=DIRECTION('ref_axis',(1.,0.,0.));
#7201=DIRECTION('center_axis',(0.,1.,0.));
#7202=DIRECTION('ref_axis',(1.,0.,0.));
#7203=DIRECTION('center_axis',(0.,-1.,0.));
#7204=DIRECTION('ref_axis',(0.,0.,-1.));
#7205=DIRECTION('center_axis',(0.,0.,1.));
#7206=DIRECTION('ref_axis',(1.,0.,0.));
#7207=DIRECTION('center_axis',(0.,-1.,0.));
#7208=DIRECTION('ref_axis',(0.,0.,-1.));
#7209=DIRECTION('center_axis',(0.,-1.,0.));
#7210=DIRECTION('ref_axis',(-1.,0.,0.));
#7211=DIRECTION('center_axis',(0.,1.,0.));
#7212=DIRECTION('ref_axis',(1.,0.,0.));
#8586=CARTESIAN_POINT('',(0.,0.,0.));
#8587=CARTESIAN_POINT('Origin',(1.18440385848747,0.,1.18440385848747));
#8588=CARTESIAN_POINT('',(0.846804978391753,-0.07938,1.40825612658882));
#8589=CARTESIAN_POINT('',(1.40825612658882,-0.07938,0.846804978391754));
#8590=CARTESIAN_POINT('Ctrl Pts',(0.846804978391752,-0.0793800000000001,
1.40825612658882));
#8591=CARTESIAN_POINT('Ctrl Pts',(0.854205272175554,-0.123401821157026,
1.40380622184538));
#8592=CARTESIAN_POINT('Ctrl Pts',(0.867957148219441,-0.166543350814306,
1.39550172959303));
#8593=CARTESIAN_POINT('Ctrl Pts',(0.902193646979982,-0.237231147975234,
1.3735491215176));
#8594=CARTESIAN_POINT('Ctrl Pts',(0.920778333482564,-0.266264900654909,
1.36127834356734));
#8595=CARTESIAN_POINT('Ctrl Pts',(0.962485392528369,-0.317195968905306,
1.33211611256184));
#8596=CARTESIAN_POINT('Ctrl Pts',(0.985600426557816,-0.33909093068465,1.31521005565926));
#8597=CARTESIAN_POINT('Ctrl Pts',(1.03253285680459,-0.373586846396559,1.27866649102984));
#8598=CARTESIAN_POINT('Ctrl Pts',(1.05871835910697,-0.388086240756494,1.25722555095714));
#8599=CARTESIAN_POINT('Ctrl Pts',(1.11153475808518,-0.407068917407805,1.2107812086231));
#8600=CARTESIAN_POINT('Ctrl Pts',(1.13814686046673,-0.411552957311693,1.18575674747573));
#8601=CARTESIAN_POINT('Ctrl Pts',(1.18575674747573,-0.411552957311693,1.13814686046673));
#8602=CARTESIAN_POINT('Ctrl Pts',(1.2107812086231,-0.407068917407805,1.11153475808518));
#8603=CARTESIAN_POINT('Ctrl Pts',(1.25722555095713,-0.388086240756494,1.05871835910697));
#8604=CARTESIAN_POINT('Ctrl Pts',(1.27866649102984,-0.373586846396559,1.03253285680459));
#8605=CARTESIAN_POINT('Ctrl Pts',(1.31521005565926,-0.33909093068465,0.985600426557816));
#8606=CARTESIAN_POINT('Ctrl Pts',(1.33211611256184,-0.317195968905306,0.962485392528369));
#8607=CARTESIAN_POINT('Ctrl Pts',(1.36127834356734,-0.266264900654909,0.920778333482565));
#8608=CARTESIAN_POINT('Ctrl Pts',(1.3735491215176,-0.237231147975234,0.902193646979983));
#8609=CARTESIAN_POINT('Ctrl Pts',(1.39550172959303,-0.166543350814306,0.867957148219442));
#8610=CARTESIAN_POINT('Ctrl Pts',(1.40380622184538,-0.123401821157026,0.854205272175555));
#8611=CARTESIAN_POINT('Ctrl Pts',(1.40825612658882,-0.0793800000000001,
0.846804978391753));
#8612=CARTESIAN_POINT('',(0.886256117232623,-0.07938,1.45861320581289));
#8613=CARTESIAN_POINT('Origin',(1.18440385848747,-0.07938,1.18440385848747));
#8614=CARTESIAN_POINT('',(1.45861320581289,-0.07938,0.886256117232624));
#8615=CARTESIAN_POINT('Ctrl Pts',(1.45861320581289,-0.0793800000000001,
0.886256117232623));
#8616=CARTESIAN_POINT('Ctrl Pts',(1.45630208793976,-0.101649918886749,0.890059788636852));
#8617=CARTESIAN_POINT('Ctrl Pts',(1.45296717977858,-0.123823518623746,0.895520212222107));
#8618=CARTESIAN_POINT('Ctrl Pts',(1.43904931717599,-0.192480977588836,0.917859913453975));
#8619=CARTESIAN_POINT('Ctrl Pts',(1.4243271592157,-0.236152929235938,0.940896403863072));
#8620=CARTESIAN_POINT('Ctrl Pts',(1.39055359345152,-0.303141259068212,0.990027513266106));
#8621=CARTESIAN_POINT('Ctrl Pts',(1.36743459453896,-0.335108247315849,1.02199477007745));
#8622=CARTESIAN_POINT('Ctrl Pts',(1.32643091652006,-0.373243761060364,1.07446535104584));
#8623=CARTESIAN_POINT('Ctrl Pts',(1.30441816675528,-0.387888272594439,1.10126842659597));
#8624=CARTESIAN_POINT('Ctrl Pts',(1.25681160160691,-0.407041111792943,1.15530234155453));
#8625=CARTESIAN_POINT('Ctrl Pts',(1.23119764287622,-0.411552957311693,1.18251418313119));
#8626=CARTESIAN_POINT('Ctrl Pts',(1.18251418313119,-0.411552957311693,1.23119764287622));
#8627=CARTESIAN_POINT('Ctrl Pts',(1.15530234155453,-0.407041111792943,1.25681160160691));
#8628=CARTESIAN_POINT('Ctrl Pts',(1.10126842659597,-0.387888272594439,1.30441816675528));
#8629=CARTESIAN_POINT('Ctrl Pts',(1.07446535104584,-0.373243761060364,1.32643091652006));
#8630=CARTESIAN_POINT('Ctrl Pts',(1.02199477007745,-0.335108247315848,1.36743459453896));
#8631=CARTESIAN_POINT('Ctrl Pts',(0.990027513266105,-0.303141259068211,
1.39055359345152));
#8632=CARTESIAN_POINT('Ctrl Pts',(0.940896403863071,-0.236152929235937,
1.42432715921571));
#8633=CARTESIAN_POINT('Ctrl Pts',(0.917859913453974,-0.192480977588835,
1.43904931717599));
#8634=CARTESIAN_POINT('Ctrl Pts',(0.895520212222106,-0.123823518623745,
1.45296717977858));
#8635=CARTESIAN_POINT('Ctrl Pts',(0.890059788636851,-0.101649918886749,
1.45630208793976));
#8636=CARTESIAN_POINT('Ctrl Pts',(0.886256117232622,-0.0793800000000001,
1.45861320581289));
#8637=CARTESIAN_POINT('Origin',(1.18440385848747,-0.07938,1.18440385848747));
#8638=CARTESIAN_POINT('Origin',(0.,-0.27783,0.));
#8639=CARTESIAN_POINT('',(0.404717578595295,-0.07938,1.65807299932179));
#8640=CARTESIAN_POINT('Origin',(0.,-0.07938,0.));
#8641=CARTESIAN_POINT('',(-0.404717578595296,-0.07938,1.65807299932179));
#8642=CARTESIAN_POINT('Ctrl Pts',(0.404717578595296,-0.0793800000000001,
1.65807299932179));
#8643=CARTESIAN_POINT('Ctrl Pts',(0.400393769631747,-0.101649918886749,
1.65912839404491));
#8644=CARTESIAN_POINT('Ctrl Pts',(0.394174530911058,-0.123823518623745,
1.66063136041479));
#8645=CARTESIAN_POINT('Ctrl Pts',(0.368536561654407,-0.192480977588835,
1.66658649961961));
#8646=CARTESIAN_POINT('Ctrl Pts',(0.341837165343982,-0.236152929235937,
1.67246562047521));
#8647=CARTESIAN_POINT('Ctrl Pts',(0.283214707341173,-0.303141259068211,
1.68332504372461));
#8648=CARTESIAN_POINT('Ctrl Pts',(0.244262842368623,-0.335108247315849,
1.68958170688653));
#8649=CARTESIAN_POINT('Ctrl Pts',(0.178166559972324,-0.373243761060364,
1.69769003172132));
#8650=CARTESIAN_POINT('Ctrl Pts',(0.143648558862931,-0.387888272594439,
1.70107730356824));
#8651=CARTESIAN_POINT('Ctrl Pts',(0.0717778861362652,-0.407041111792943,
1.70562212620408));
#8652=CARTESIAN_POINT('Ctrl Pts',(0.0344244045173309,-0.411552957311693,
1.706752));
#8653=CARTESIAN_POINT('Ctrl Pts',(-0.0344244045173315,-0.411552957311693,
1.706752));
#8654=CARTESIAN_POINT('Ctrl Pts',(-0.0717778861362658,-0.407041111792943,
1.70562212620408));
#8655=CARTESIAN_POINT('Ctrl Pts',(-0.143648558862932,-0.387888272594439,
1.70107730356824));
#8656=CARTESIAN_POINT('Ctrl Pts',(-0.178166559972325,-0.373243761060364,
1.69769003172132));
#8657=CARTESIAN_POINT('Ctrl Pts',(-0.244262842368624,-0.335108247315849,
1.68958170688653));
#8658=CARTESIAN_POINT('Ctrl Pts',(-0.283214707341173,-0.303141259068212,
1.68332504372461));
#8659=CARTESIAN_POINT('Ctrl Pts',(-0.341837165343982,-0.236152929235937,
1.67246562047521));
#8660=CARTESIAN_POINT('Ctrl Pts',(-0.368536561654408,-0.192480977588835,
1.66658649961961));
#8661=CARTESIAN_POINT('Ctrl Pts',(-0.394174530911059,-0.123823518623745,
1.66063136041479));
#8662=CARTESIAN_POINT('Ctrl Pts',(-0.400393769631748,-0.101649918886749,
1.65912839404491));
#8663=CARTESIAN_POINT('Ctrl Pts',(-0.404717578595297,-0.0793800000000001,
1.65807299932179));
#8664=CARTESIAN_POINT('',(-0.886256117232624,-0.07938,1.45861320581289));
#8665=CARTESIAN_POINT('Origin',(0.,-0.07938,0.));
#8666=CARTESIAN_POINT('',(-1.45861320581289,-0.07938,0.886256117232623));
#8667=CARTESIAN_POINT('Ctrl Pts',(-0.886256117232623,-0.0793800000000001,
1.45861320581289));
#8668=CARTESIAN_POINT('Ctrl Pts',(-0.890059788636852,-0.101649918886749,
1.45630208793976));
#8669=CARTESIAN_POINT('Ctrl Pts',(-0.895520212222106,-0.123823518623745,
1.45296717977858));
#8670=CARTESIAN_POINT('Ctrl Pts',(-0.917859913453974,-0.192480977588835,
1.43904931717599));
#8671=CARTESIAN_POINT('Ctrl Pts',(-0.940896403863071,-0.236152929235937,
1.4243271592157));
#8672=CARTESIAN_POINT('Ctrl Pts',(-0.990027513266105,-0.303141259068211,
1.39055359345152));
#8673=CARTESIAN_POINT('Ctrl Pts',(-1.02199477007745,-0.335108247315848,
1.36743459453896));
#8674=CARTESIAN_POINT('Ctrl Pts',(-1.07446535104584,-0.373243761060364,
1.32643091652006));
#8675=CARTESIAN_POINT('Ctrl Pts',(-1.10126842659597,-0.387888272594439,
1.30441816675528));
#8676=CARTESIAN_POINT('Ctrl Pts',(-1.15530234155453,-0.407041111792943,
1.25681160160691));
#8677=CARTESIAN_POINT('Ctrl Pts',(-1.18251418313119,-0.411552957311693,
1.23119764287622));
#8678=CARTESIAN_POINT('Ctrl Pts',(-1.23119764287622,-0.411552957311693,
1.18251418313119));
#8679=CARTESIAN_POINT('Ctrl Pts',(-1.25681160160691,-0.407041111792943,
1.15530234155453));
#8680=CARTESIAN_POINT('Ctrl Pts',(-1.30441816675528,-0.387888272594439,
1.10126842659597));
#8681=CARTESIAN_POINT('Ctrl Pts',(-1.32643091652006,-0.373243761060365,
1.07446535104584));
#8682=CARTESIAN_POINT('Ctrl Pts',(-1.36743459453896,-0.335108247315849,
1.02199477007745));
#8683=CARTESIAN_POINT('Ctrl Pts',(-1.39055359345152,-0.303141259068212,
0.990027513266106));
#8684=CARTESIAN_POINT('Ctrl Pts',(-1.4243271592157,-0.236152929235938,0.940896403863071));
#8685=CARTESIAN_POINT('Ctrl Pts',(-1.43904931717599,-0.192480977588836,
0.917859913453974));
#8686=CARTESIAN_POINT('Ctrl Pts',(-1.45296717977858,-0.123823518623746,
0.895520212222106));
#8687=CARTESIAN_POINT('Ctrl Pts',(-1.45630208793976,-0.101649918886749,
0.890059788636852));
#8688=CARTESIAN_POINT('Ctrl Pts',(-1.45861320581289,-0.0793800000000001,
0.886256117232623));
#8689=CARTESIAN_POINT('',(-1.65807299932179,-0.07938,0.404717578595295));
#8690=CARTESIAN_POINT('Origin',(0.,-0.07938,0.));
#8691=CARTESIAN_POINT('',(-1.706752,-0.411552957311693,2.08591827245526E-16));
#8692=CARTESIAN_POINT('Ctrl Pts',(-1.65807299932179,-0.0793800000000001,
0.404717578595296));
#8693=CARTESIAN_POINT('Ctrl Pts',(-1.65912839404491,-0.101649918886749,
0.400393769631747));
#8694=CARTESIAN_POINT('Ctrl Pts',(-1.66063136041479,-0.123823518623745,
0.394174530911058));
#8695=CARTESIAN_POINT('Ctrl Pts',(-1.66658649961961,-0.192480977588835,
0.368536561654407));
#8696=CARTESIAN_POINT('Ctrl Pts',(-1.67246562047521,-0.236152929235937,
0.341837165343982));
#8697=CARTESIAN_POINT('Ctrl Pts',(-1.68332504372461,-0.303141259068211,
0.283214707341173));
#8698=CARTESIAN_POINT('Ctrl Pts',(-1.68958170688653,-0.335108247315848,
0.244262842368623));
#8699=CARTESIAN_POINT('Ctrl Pts',(-1.69769003172132,-0.373243761060364,
0.178166559972324));
#8700=CARTESIAN_POINT('Ctrl Pts',(-1.70107730356824,-0.387888272594439,
0.143648558862931));
#8701=CARTESIAN_POINT('Ctrl Pts',(-1.70562212620408,-0.407041111792943,
0.0717778861362656));
#8702=CARTESIAN_POINT('Ctrl Pts',(-1.706752,-0.411552957311693,0.0344244045173313));
#8703=CARTESIAN_POINT('Ctrl Pts',(-1.706752,-0.411552957311693,2.08166817117217E-16));
#8704=CARTESIAN_POINT('',(-1.706752,-0.47628,2.09016837373834E-16));
#8705=CARTESIAN_POINT('',(-1.706752,-0.27783,2.09016837373834E-16));
#8706=CARTESIAN_POINT('Origin',(0.,-0.47628,0.));
#8707=CARTESIAN_POINT('',(-1.65807299932179,-0.07938,-0.404717578595296));
#8708=CARTESIAN_POINT('Ctrl Pts',(-1.706752,-0.411552957311693,2.0122792321331E-16));
#8709=CARTESIAN_POINT('Ctrl Pts',(-1.706752,-0.411552957311693,-0.0344244045173309));
#8710=CARTESIAN_POINT('Ctrl Pts',(-1.70562212620408,-0.407041111792943,
-0.0717778861362652));
#8711=CARTESIAN_POINT('Ctrl Pts',(-1.70107730356824,-0.387888272594439,
-0.143648558862931));
#8712=CARTESIAN_POINT('Ctrl Pts',(-1.69769003172132,-0.373243761060365,
-0.178166559972324));
#8713=CARTESIAN_POINT('Ctrl Pts',(-1.68958170688653,-0.335108247315849,
-0.244262842368623));
#8714=CARTESIAN_POINT('Ctrl Pts',(-1.68332504372461,-0.303141259068212,
-0.283214707341173));
#8715=CARTESIAN_POINT('Ctrl Pts',(-1.67246562047521,-0.236152929235938,
-0.341837165343982));
#8716=CARTESIAN_POINT('Ctrl Pts',(-1.66658649961961,-0.192480977588836,
-0.368536561654407));
#8717=CARTESIAN_POINT('Ctrl Pts',(-1.66063136041479,-0.123823518623745,
-0.394174530911059));
#8718=CARTESIAN_POINT('Ctrl Pts',(-1.65912839404491,-0.101649918886749,
-0.400393769631748));
#8719=CARTESIAN_POINT('Ctrl Pts',(-1.65807299932179,-0.0793800000000001,
-0.404717578595296));
#8720=CARTESIAN_POINT('',(-1.45861320581289,-0.07938,-0.886256117232623));
#8721=CARTESIAN_POINT('Origin',(0.,-0.07938,0.));
#8722=CARTESIAN_POINT('',(-0.886256117232623,-0.07938,-1.45861320581289));
#8723=CARTESIAN_POINT('Ctrl Pts',(-1.45861320581289,-0.0793800000000001,
-0.886256117232623));
#8724=CARTESIAN_POINT('Ctrl Pts',(-1.45630208793976,-0.101649918886749,
-0.890059788636852));
#8725=CARTESIAN_POINT('Ctrl Pts',(-1.45296717977858,-0.123823518623745,
-0.895520212222106));
#8726=CARTESIAN_POINT('Ctrl Pts',(-1.43904931717599,-0.192480977588835,
-0.917859913453974));
#8727=CARTESIAN_POINT('Ctrl Pts',(-1.4243271592157,-0.236152929235937,-0.940896403863072));
#8728=CARTESIAN_POINT('Ctrl Pts',(-1.39055359345152,-0.303141259068212,
-0.990027513266106));
#8729=CARTESIAN_POINT('Ctrl Pts',(-1.36743459453896,-0.335108247315849,
-1.02199477007745));
#8730=CARTESIAN_POINT('Ctrl Pts',(-1.32643091652006,-0.373243761060364,
-1.07446535104584));
#8731=CARTESIAN_POINT('Ctrl Pts',(-1.30441816675528,-0.387888272594439,
-1.10126842659597));
#8732=CARTESIAN_POINT('Ctrl Pts',(-1.25681160160691,-0.407041111792943,
-1.15530234155453));
#8733=CARTESIAN_POINT('Ctrl Pts',(-1.23119764287622,-0.411552957311693,
-1.18251418313119));
#8734=CARTESIAN_POINT('Ctrl Pts',(-1.18251418313119,-0.411552957311693,
-1.23119764287622));
#8735=CARTESIAN_POINT('Ctrl Pts',(-1.15530234155453,-0.407041111792943,
-1.25681160160691));
#8736=CARTESIAN_POINT('Ctrl Pts',(-1.10126842659597,-0.387888272594439,
-1.30441816675528));
#8737=CARTESIAN_POINT('Ctrl Pts',(-1.07446535104584,-0.373243761060364,
-1.32643091652006));
#8738=CARTESIAN_POINT('Ctrl Pts',(-1.02199477007745,-0.335108247315848,
-1.36743459453896));
#8739=CARTESIAN_POINT('Ctrl Pts',(-0.990027513266105,-0.303141259068211,
-1.39055359345152));
#8740=CARTESIAN_POINT('Ctrl Pts',(-0.940896403863071,-0.236152929235936,
-1.42432715921571));
#8741=CARTESIAN_POINT('Ctrl Pts',(-0.917859913453974,-0.192480977588835,
-1.43904931717599));
#8742=CARTESIAN_POINT('Ctrl Pts',(-0.895520212222106,-0.123823518623745,
-1.45296717977858));
#8743=CARTESIAN_POINT('Ctrl Pts',(-0.890059788636851,-0.101649918886749,
-1.45630208793976));
#8744=CARTESIAN_POINT('Ctrl Pts',(-0.886256117232623,-0.0793800000000001,
-1.45861320581289));
#8745=CARTESIAN_POINT('',(-0.404717578595295,-0.07938,-1.65807299932179));
#8746=CARTESIAN_POINT('Origin',(0.,-0.07938,0.));
#8747=CARTESIAN_POINT('',(0.404717578595296,-0.07938,-1.65807299932179));
#8748=CARTESIAN_POINT('Ctrl Pts',(-0.404717578595296,-0.0793800000000001,
-1.65807299932179));
#8749=CARTESIAN_POINT('Ctrl Pts',(-0.400393769631747,-0.101649918886749,
-1.65912839404491));
#8750=CARTESIAN_POINT('Ctrl Pts',(-0.394174530911058,-0.123823518623746,
-1.66063136041479));
#8751=CARTESIAN_POINT('Ctrl Pts',(-0.368536561654407,-0.192480977588836,
-1.66658649961961));
#8752=CARTESIAN_POINT('Ctrl Pts',(-0.341837165343982,-0.236152929235938,
-1.67246562047521));
#8753=CARTESIAN_POINT('Ctrl Pts',(-0.283214707341173,-0.303141259068212,
-1.68332504372461));
#8754=CARTESIAN_POINT('Ctrl Pts',(-0.244262842368623,-0.335108247315849,
-1.68958170688653));
#8755=CARTESIAN_POINT('Ctrl Pts',(-0.178166559972324,-0.373243761060364,
-1.69769003172132));
#8756=CARTESIAN_POINT('Ctrl Pts',(-0.143648558862931,-0.387888272594439,
-1.70107730356824));
#8757=CARTESIAN_POINT('Ctrl Pts',(-0.0717778861362653,-0.407041111792943,
-1.70562212620408));
#8758=CARTESIAN_POINT('Ctrl Pts',(-0.034424404517331,-0.411552957311693,
-1.706752));
#8759=CARTESIAN_POINT('Ctrl Pts',(0.0344244045173312,-0.411552957311693,
-1.706752));
#8760=CARTESIAN_POINT('Ctrl Pts',(0.0717778861362655,-0.407041111792943,
-1.70562212620408));
#8761=CARTESIAN_POINT('Ctrl Pts',(0.143648558862931,-0.387888272594439,
-1.70107730356824));
#8762=CARTESIAN_POINT('Ctrl Pts',(0.178166559972324,-0.373243761060364,
-1.69769003172132));
#8763=CARTESIAN_POINT('Ctrl Pts',(0.244262842368623,-0.335108247315849,
-1.68958170688653));
#8764=CARTESIAN_POINT('Ctrl Pts',(0.283214707341173,-0.303141259068212,
-1.68332504372461));
#8765=CARTESIAN_POINT('Ctrl Pts',(0.341837165343982,-0.236152929235937,
-1.67246562047521));
#8766=CARTESIAN_POINT('Ctrl Pts',(0.368536561654407,-0.192480977588835,
-1.66658649961961));
#8767=CARTESIAN_POINT('Ctrl Pts',(0.394174530911059,-0.123823518623745,
-1.66063136041479));
#8768=CARTESIAN_POINT('Ctrl Pts',(0.400393769631748,-0.101649918886749,
-1.65912839404491));
#8769=CARTESIAN_POINT('Ctrl Pts',(0.404717578595296,-0.0793800000000001,
-1.65807299932179));
#8770=CARTESIAN_POINT('',(0.886256117232623,-0.07938,-1.45861320581289));
#8771=CARTESIAN_POINT('Origin',(0.,-0.07938,0.));
#8772=CARTESIAN_POINT('',(1.45861320581289,-0.07938,-0.886256117232623));
#8773=CARTESIAN_POINT('Ctrl Pts',(0.886256117232623,-0.0793800000000001,
-1.45861320581289));
#8774=CARTESIAN_POINT('Ctrl Pts',(0.890059788636852,-0.101649918886749,
-1.45630208793976));
#8775=CARTESIAN_POINT('Ctrl Pts',(0.895520212222106,-0.123823518623745,
-1.45296717977858));
#8776=CARTESIAN_POINT('Ctrl Pts',(0.917859913453974,-0.192480977588835,
-1.43904931717599));
#8777=CARTESIAN_POINT('Ctrl Pts',(0.940896403863072,-0.236152929235937,
-1.4243271592157));
#8778=CARTESIAN_POINT('Ctrl Pts',(0.990027513266106,-0.303141259068211,
-1.39055359345152));
#8779=CARTESIAN_POINT('Ctrl Pts',(1.02199477007745,-0.335108247315849,-1.36743459453896));
#8780=CARTESIAN_POINT('Ctrl Pts',(1.07446535104584,-0.373243761060364,-1.32643091652006));
#8781=CARTESIAN_POINT('Ctrl Pts',(1.10126842659597,-0.387888272594439,-1.30441816675528));
#8782=CARTESIAN_POINT('Ctrl Pts',(1.15530234155453,-0.407041111792943,-1.25681160160691));
#8783=CARTESIAN_POINT('Ctrl Pts',(1.18251418313119,-0.411552957311693,-1.23119764287622));
#8784=CARTESIAN_POINT('Ctrl Pts',(1.23119764287622,-0.411552957311693,-1.18251418313119));
#8785=CARTESIAN_POINT('Ctrl Pts',(1.25681160160691,-0.407041111792943,-1.15530234155453));
#8786=CARTESIAN_POINT('Ctrl Pts',(1.30441816675528,-0.387888272594439,-1.10126842659597));
#8787=CARTESIAN_POINT('Ctrl Pts',(1.32643091652006,-0.373243761060364,-1.07446535104584));
#8788=CARTESIAN_POINT('Ctrl Pts',(1.36743459453896,-0.335108247315849,-1.02199477007745));
#8789=CARTESIAN_POINT('Ctrl Pts',(1.39055359345152,-0.303141259068212,-0.990027513266105));
#8790=CARTESIAN_POINT('Ctrl Pts',(1.4243271592157,-0.236152929235937,-0.940896403863071));
#8791=CARTESIAN_POINT('Ctrl Pts',(1.43904931717599,-0.192480977588835,-0.917859913453974));
#8792=CARTESIAN_POINT('Ctrl Pts',(1.45296717977858,-0.123823518623745,-0.895520212222106));
#8793=CARTESIAN_POINT('Ctrl Pts',(1.45630208793976,-0.101649918886749,-0.890059788636852));
#8794=CARTESIAN_POINT('Ctrl Pts',(1.45861320581289,-0.0793800000000001,
-0.886256117232623));
#8795=CARTESIAN_POINT('',(1.65807299932179,-0.07938,-0.404717578595296));
#8796=CARTESIAN_POINT('Origin',(0.,-0.07938,0.));
#8797=CARTESIAN_POINT('',(1.65807299932179,-0.07938,0.404717578595296));
#8798=CARTESIAN_POINT('Ctrl Pts',(1.65807299932179,-0.0793800000000001,
-0.404717578595296));
#8799=CARTESIAN_POINT('Ctrl Pts',(1.65912839404491,-0.101649918886749,-0.400393769631747));
#8800=CARTESIAN_POINT('Ctrl Pts',(1.66063136041479,-0.123823518623745,-0.394174530911058));
#8801=CARTESIAN_POINT('Ctrl Pts',(1.66658649961961,-0.192480977588835,-0.368536561654407));
#8802=CARTESIAN_POINT('Ctrl Pts',(1.67246562047521,-0.236152929235937,-0.341837165343982));
#8803=CARTESIAN_POINT('Ctrl Pts',(1.68332504372461,-0.303141259068212,-0.283214707341173));
#8804=CARTESIAN_POINT('Ctrl Pts',(1.68958170688653,-0.335108247315849,-0.244262842368623));
#8805=CARTESIAN_POINT('Ctrl Pts',(1.69769003172132,-0.373243761060364,-0.178166559972324));
#8806=CARTESIAN_POINT('Ctrl Pts',(1.70107730356824,-0.387888272594439,-0.143648558862931));
#8807=CARTESIAN_POINT('Ctrl Pts',(1.70562212620408,-0.407041111792943,-0.0717778861362655));
#8808=CARTESIAN_POINT('Ctrl Pts',(1.706752,-0.411552957311693,-0.0344244045173312));
#8809=CARTESIAN_POINT('Ctrl Pts',(1.706752,-0.411552957311693,0.0344244045173312));
#8810=CARTESIAN_POINT('Ctrl Pts',(1.70562212620408,-0.407041111792943,0.0717778861362655));
#8811=CARTESIAN_POINT('Ctrl Pts',(1.70107730356824,-0.387888272594439,0.143648558862931));
#8812=CARTESIAN_POINT('Ctrl Pts',(1.69769003172132,-0.373243761060364,0.178166559972324));
#8813=CARTESIAN_POINT('Ctrl Pts',(1.68958170688653,-0.335108247315849,0.244262842368623));
#8814=CARTESIAN_POINT('Ctrl Pts',(1.68332504372461,-0.303141259068212,0.283214707341173));
#8815=CARTESIAN_POINT('Ctrl Pts',(1.67246562047521,-0.236152929235937,0.341837165343982));
#8816=CARTESIAN_POINT('Ctrl Pts',(1.66658649961961,-0.192480977588835,0.368536561654407));
#8817=CARTESIAN_POINT('Ctrl Pts',(1.66063136041479,-0.123823518623745,0.394174530911058));
#8818=CARTESIAN_POINT('Ctrl Pts',(1.65912839404491,-0.101649918886749,0.400393769631747));
#8819=CARTESIAN_POINT('Ctrl Pts',(1.65807299932179,-0.0793800000000001,
0.404717578595296));
#8820=CARTESIAN_POINT('Origin',(0.,-0.07938,0.));
#8821=CARTESIAN_POINT('Origin',(0.,-0.07938,0.));
#8822=CARTESIAN_POINT('',(0.397005914195118,-0.07938,1.59456899932179));
#8823=CARTESIAN_POINT('Origin',(0.,-0.07938,0.));
#8824=CARTESIAN_POINT('Origin',(-3.33066907387547E-16,-0.07938,1.675));
#8825=CARTESIAN_POINT('Origin',(-3.33066907387547E-16,0.,1.675));
#8826=CARTESIAN_POINT('',(-0.397005914195118,-0.07938,1.59456899932179));
#8827=CARTESIAN_POINT('Ctrl Pts',(-0.397005914195119,-0.0793800000000001,
1.59456899932179));
#8828=CARTESIAN_POINT('Ctrl Pts',(-0.3886265584581,-0.123401821157026,1.59665523941937));
#8829=CARTESIAN_POINT('Ctrl Pts',(-0.373030350867485,-0.166543350814306,
1.60050712143809));
#8830=CARTESIAN_POINT('Ctrl Pts',(-0.333298652394954,-0.237231147975234,
1.60919314384089));
#8831=CARTESIAN_POINT('Ctrl Pts',(-0.311480544243687,-0.266264900654909,
1.61365775139403));
#8832=CARTESIAN_POINT('Ctrl Pts',(-0.261368388670537,-0.317195968905306,
1.62252828437015));
#8833=CARTESIAN_POINT('Ctrl Pts',(-0.233069203882014,-0.33909093068465,
1.62691869420078));
#8834=CARTESIAN_POINT('Ctrl Pts',(-0.174042761838764,-0.373586846396559,
1.63426473152765));
#8835=CARTESIAN_POINT('Ctrl Pts',(-0.14036578147155,-0.388086240756494,
1.63761964365402));
#8836=CARTESIAN_POINT('Ctrl Pts',(-0.0701778381840615,-0.407068917407805,
1.64212536811722));
#8837=CARTESIAN_POINT('Ctrl Pts',(-0.0336652739555918,-0.411552957311693,
1.643248));
#8838=CARTESIAN_POINT('Ctrl Pts',(0.0336652739555913,-0.411552957311693,
1.643248));
#8839=CARTESIAN_POINT('Ctrl Pts',(0.070177838184061,-0.407068917407805,
1.64212536811722));
#8840=CARTESIAN_POINT('Ctrl Pts',(0.140365781471549,-0.388086240756494,
1.63761964365402));
#8841=CARTESIAN_POINT('Ctrl Pts',(0.174042761838763,-0.373586846396559,
1.63426473152765));
#8842=CARTESIAN_POINT('Ctrl Pts',(0.233069203882014,-0.33909093068465,1.62691869420078));
#8843=CARTESIAN_POINT('Ctrl Pts',(0.261368388670536,-0.317195968905306,
1.62252828437015));
#8844=CARTESIAN_POINT('Ctrl Pts',(0.311480544243686,-0.266264900654908,
1.61365775139403));
#8845=CARTESIAN_POINT('Ctrl Pts',(0.333298652394954,-0.237231147975234,
1.60919314384089));
#8846=CARTESIAN_POINT('Ctrl Pts',(0.373030350867484,-0.166543350814306,
1.60050712143809));
#8847=CARTESIAN_POINT('Ctrl Pts',(0.388626558458099,-0.123401821157026,
1.59665523941937));
#8848=CARTESIAN_POINT('Ctrl Pts',(0.397005914195118,-0.07938,1.59456899932179));
#8849=CARTESIAN_POINT('Origin',(-3.33066907387547E-16,-0.07938,1.675));
#8850=CARTESIAN_POINT('Origin',(0.,-0.07938,0.));
#8851=CARTESIAN_POINT('',(-0.846804978391754,-0.07938,1.40825612658882));
#8852=CARTESIAN_POINT('Origin',(0.,-0.07938,0.));
#8853=CARTESIAN_POINT('Origin',(-1.18440385848747,-0.07938,1.18440385848747));
#8854=CARTESIAN_POINT('Origin',(-1.18440385848747,0.,1.18440385848747));
#8855=CARTESIAN_POINT('',(-1.40825612658882,-0.07938,0.846804978391753));
#8856=CARTESIAN_POINT('Ctrl Pts',(-1.40825612658882,-0.0793800000000001,
0.846804978391753));
#8857=CARTESIAN_POINT('Ctrl Pts',(-1.40380622184538,-0.123401821157026,
0.854205272175555));
#8858=CARTESIAN_POINT('Ctrl Pts',(-1.39550172959303,-0.166543350814306,
0.867957148219442));
#8859=CARTESIAN_POINT('Ctrl Pts',(-1.3735491215176,-0.237231147975235,0.902193646979983));
#8860=CARTESIAN_POINT('Ctrl Pts',(-1.36127834356734,-0.266264900654909,
0.920778333482565));
#8861=CARTESIAN_POINT('Ctrl Pts',(-1.33211611256184,-0.317195968905306,
0.962485392528369));
#8862=CARTESIAN_POINT('Ctrl Pts',(-1.31521005565926,-0.339090930684651,
0.985600426557816));
#8863=CARTESIAN_POINT('Ctrl Pts',(-1.27866649102984,-0.373586846396559,
1.03253285680459));
#8864=CARTESIAN_POINT('Ctrl Pts',(-1.25722555095714,-0.388086240756494,
1.05871835910697));
#8865=CARTESIAN_POINT('Ctrl Pts',(-1.2107812086231,-0.407068917407805,1.11153475808518));
#8866=CARTESIAN_POINT('Ctrl Pts',(-1.18575674747573,-0.411552957311693,
1.13814686046673));
#8867=CARTESIAN_POINT('Ctrl Pts',(-1.13814686046673,-0.411552957311693,
1.18575674747573));
#8868=CARTESIAN_POINT('Ctrl Pts',(-1.11153475808518,-0.407068917407805,
1.2107812086231));
#8869=CARTESIAN_POINT('Ctrl Pts',(-1.05871835910697,-0.388086240756494,
1.25722555095714));
#8870=CARTESIAN_POINT('Ctrl Pts',(-1.03253285680459,-0.373586846396559,
1.27866649102984));
#8871=CARTESIAN_POINT('Ctrl Pts',(-0.985600426557816,-0.33909093068465,
1.31521005565926));
#8872=CARTESIAN_POINT('Ctrl Pts',(-0.962485392528369,-0.317195968905306,
1.33211611256184));
#8873=CARTESIAN_POINT('Ctrl Pts',(-0.920778333482565,-0.266264900654908,
1.36127834356734));
#8874=CARTESIAN_POINT('Ctrl Pts',(-0.902193646979983,-0.237231147975234,
1.3735491215176));
#8875=CARTESIAN_POINT('Ctrl Pts',(-0.867957148219442,-0.166543350814306,
1.39550172959303));
#8876=CARTESIAN_POINT('Ctrl Pts',(-0.854205272175555,-0.123401821157026,
1.40380622184538));
#8877=CARTESIAN_POINT('Ctrl Pts',(-0.846804978391753,-0.0793800000000001,
1.40825612658882));
#8878=CARTESIAN_POINT('Origin',(-1.18440385848747,-0.07938,1.18440385848747));
#8879=CARTESIAN_POINT('Origin',(0.,-0.07938,0.));
#8880=CARTESIAN_POINT('',(-1.59456899932179,-0.07938,0.397005914195118));
#8881=CARTESIAN_POINT('Origin',(0.,-0.07938,0.));
#8882=CARTESIAN_POINT('Origin',(-1.675,-0.07938,-2.22044604925031E-16));
#8883=CARTESIAN_POINT('Origin',(-1.675,0.,-2.22044604925031E-16));
#8884=CARTESIAN_POINT('',(-1.59456899932179,-0.07938,-0.397005914195118));
#8885=CARTESIAN_POINT('',(-1.643248,-0.411552957311693,3.47540551556327E-18));
#8886=CARTESIAN_POINT('Ctrl Pts',(-1.59456899932179,-0.0793800000000001,
-0.397005914195119));
#8887=CARTESIAN_POINT('Ctrl Pts',(-1.59665523941937,-0.123401821157026,
-0.388626558458099));
#8888=CARTESIAN_POINT('Ctrl Pts',(-1.60050712143809,-0.166543350814306,
-0.373030350867485));
#8889=CARTESIAN_POINT('Ctrl Pts',(-1.60919314384089,-0.237231147975234,
-0.333298652394954));
#8890=CARTESIAN_POINT('Ctrl Pts',(-1.61365775139403,-0.266264900654909,
-0.311480544243686));
#8891=CARTESIAN_POINT('Ctrl Pts',(-1.62252828437015,-0.317195968905306,
-0.261368388670537));
#8892=CARTESIAN_POINT('Ctrl Pts',(-1.62691869420078,-0.33909093068465,-0.233069203882014));
#8893=CARTESIAN_POINT('Ctrl Pts',(-1.63426473152765,-0.373586846396559,
-0.174042761838764));
#8894=CARTESIAN_POINT('Ctrl Pts',(-1.63761964365402,-0.388086240756494,
-0.140365781471549));
#8895=CARTESIAN_POINT('Ctrl Pts',(-1.64212536811722,-0.407068917407805,
-0.0701778381840614));
#8896=CARTESIAN_POINT('Ctrl Pts',(-1.643248,-0.411552957311693,-0.0336652739555917));
#8897=CARTESIAN_POINT('Ctrl Pts',(-1.643248,-0.411552957311693,-2.0122792321331E-16));
#8898=CARTESIAN_POINT('Origin',(-1.675,-0.07938,-2.22044604925031E-16));
#8899=CARTESIAN_POINT('Ctrl Pts',(-1.643248,-0.411552957311693,-1.94289029309402E-16));
#8900=CARTESIAN_POINT('Ctrl Pts',(-1.643248,-0.411552957311693,0.0336652739555913));
#8901=CARTESIAN_POINT('Ctrl Pts',(-1.64212536811722,-0.407068917407805,
0.0701778381840609));
#8902=CARTESIAN_POINT('Ctrl Pts',(-1.63761964365402,-0.388086240756494,
0.140365781471549));
#8903=CARTESIAN_POINT('Ctrl Pts',(-1.63426473152765,-0.373586846396559,
0.174042761838763));
#8904=CARTESIAN_POINT('Ctrl Pts',(-1.62691869420078,-0.33909093068465,0.233069203882014));
#8905=CARTESIAN_POINT('Ctrl Pts',(-1.62252828437015,-0.317195968905306,
0.261368388670536));
#8906=CARTESIAN_POINT('Ctrl Pts',(-1.61365775139403,-0.266264900654909,
0.311480544243686));
#8907=CARTESIAN_POINT('Ctrl Pts',(-1.60919314384089,-0.237231147975235,
0.333298652394954));
#8908=CARTESIAN_POINT('Ctrl Pts',(-1.60050712143809,-0.166543350814306,
0.373030350867484));
#8909=CARTESIAN_POINT('Ctrl Pts',(-1.59665523941937,-0.123401821157026,
0.388626558458099));
#8910=CARTESIAN_POINT('Ctrl Pts',(-1.59456899932179,-0.0793800000000001,
0.397005914195118));
#8911=CARTESIAN_POINT('Origin',(0.,-0.07938,0.));
#8912=CARTESIAN_POINT('',(-1.40825612658882,-0.07938,-0.846804978391753));
#8913=CARTESIAN_POINT('Origin',(0.,-0.07938,0.));
#8914=CARTESIAN_POINT('Origin',(-1.18440385848747,-0.07938,-1.18440385848747));
#8915=CARTESIAN_POINT('Origin',(-1.18440385848747,0.,-1.18440385848747));
#8916=CARTESIAN_POINT('',(-0.846804978391753,-0.07938,-1.40825612658882));
#8917=CARTESIAN_POINT('Ctrl Pts',(-0.846804978391753,-0.0793800000000001,
-1.40825612658882));
#8918=CARTESIAN_POINT('Ctrl Pts',(-0.854205272175555,-0.123401821157026,
-1.40380622184538));
#8919=CARTESIAN_POINT('Ctrl Pts',(-0.867957148219442,-0.166543350814306,
-1.39550172959303));
#8920=CARTESIAN_POINT('Ctrl Pts',(-0.902193646979982,-0.237231147975234,
-1.3735491215176));
#8921=CARTESIAN_POINT('Ctrl Pts',(-0.920778333482564,-0.266264900654908,
-1.36127834356734));
#8922=CARTESIAN_POINT('Ctrl Pts',(-0.962485392528368,-0.317195968905306,
-1.33211611256184));
#8923=CARTESIAN_POINT('Ctrl Pts',(-0.985600426557816,-0.33909093068465,
-1.31521005565926));
#8924=CARTESIAN_POINT('Ctrl Pts',(-1.03253285680459,-0.373586846396559,
-1.27866649102984));
#8925=CARTESIAN_POINT('Ctrl Pts',(-1.05871835910697,-0.388086240756494,
-1.25722555095714));
#8926=CARTESIAN_POINT('Ctrl Pts',(-1.11153475808518,-0.407068917407805,
-1.2107812086231));
#8927=CARTESIAN_POINT('Ctrl Pts',(-1.13814686046673,-0.411552957311693,
-1.18575674747573));
#8928=CARTESIAN_POINT('Ctrl Pts',(-1.18575674747573,-0.411552957311693,
-1.13814686046673));
#8929=CARTESIAN_POINT('Ctrl Pts',(-1.2107812086231,-0.407068917407805,-1.11153475808518));
#8930=CARTESIAN_POINT('Ctrl Pts',(-1.25722555095714,-0.388086240756494,
-1.05871835910697));
#8931=CARTESIAN_POINT('Ctrl Pts',(-1.27866649102984,-0.373586846396559,
-1.03253285680459));
#8932=CARTESIAN_POINT('Ctrl Pts',(-1.31521005565926,-0.33909093068465,-0.985600426557816));
#8933=CARTESIAN_POINT('Ctrl Pts',(-1.33211611256184,-0.317195968905306,
-0.962485392528369));
#8934=CARTESIAN_POINT('Ctrl Pts',(-1.36127834356734,-0.266264900654909,
-0.920778333482565));
#8935=CARTESIAN_POINT('Ctrl Pts',(-1.3735491215176,-0.237231147975234,-0.902193646979983));
#8936=CARTESIAN_POINT('Ctrl Pts',(-1.39550172959303,-0.166543350814306,
-0.867957148219442));
#8937=CARTESIAN_POINT('Ctrl Pts',(-1.40380622184538,-0.123401821157026,
-0.854205272175555));
#8938=CARTESIAN_POINT('Ctrl Pts',(-1.40825612658882,-0.07938,-0.846804978391753));
#8939=CARTESIAN_POINT('Origin',(-1.18440385848747,-0.07938,-1.18440385848747));
#8940=CARTESIAN_POINT('Origin',(0.,-0.07938,0.));
#8941=CARTESIAN_POINT('',(-0.397005914195118,-0.07938,-1.59456899932179));
#8942=CARTESIAN_POINT('Origin',(0.,-0.07938,0.));
#8943=CARTESIAN_POINT('Origin',(1.11022302462516E-16,-0.07938,-1.675));
#8944=CARTESIAN_POINT('Origin',(1.11022302462516E-16,0.,-1.675));
#8945=CARTESIAN_POINT('',(0.397005914195118,-0.07938,-1.59456899932179));
#8946=CARTESIAN_POINT('Ctrl Pts',(0.397005914195119,-0.0793800000000001,
-1.59456899932179));
#8947=CARTESIAN_POINT('Ctrl Pts',(0.388626558458099,-0.123401821157026,
-1.59665523941937));
#8948=CARTESIAN_POINT('Ctrl Pts',(0.373030350867485,-0.166543350814306,
-1.60050712143809));
#8949=CARTESIAN_POINT('Ctrl Pts',(0.333298652394954,-0.237231147975234,
-1.60919314384089));
#8950=CARTESIAN_POINT('Ctrl Pts',(0.311480544243686,-0.266264900654909,
-1.61365775139403));
#8951=CARTESIAN_POINT('Ctrl Pts',(0.261368388670537,-0.317195968905306,
-1.62252828437015));
#8952=CARTESIAN_POINT('Ctrl Pts',(0.233069203882014,-0.33909093068465,-1.62691869420078));
#8953=CARTESIAN_POINT('Ctrl Pts',(0.174042761838763,-0.373586846396559,
-1.63426473152765));
#8954=CARTESIAN_POINT('Ctrl Pts',(0.140365781471549,-0.388086240756494,
-1.63761964365402));
#8955=CARTESIAN_POINT('Ctrl Pts',(0.0701778381840612,-0.407068917407805,
-1.64212536811722));
#8956=CARTESIAN_POINT('Ctrl Pts',(0.0336652739555916,-0.411552957311693,
-1.643248));
#8957=CARTESIAN_POINT('Ctrl Pts',(-0.0336652739555915,-0.411552957311693,
-1.643248));
#8958=CARTESIAN_POINT('Ctrl Pts',(-0.0701778381840612,-0.407068917407805,
-1.64212536811722));
#8959=CARTESIAN_POINT('Ctrl Pts',(-0.140365781471549,-0.388086240756494,
-1.63761964365402));
#8960=CARTESIAN_POINT('Ctrl Pts',(-0.174042761838764,-0.373586846396559,
-1.63426473152765));
#8961=CARTESIAN_POINT('Ctrl Pts',(-0.233069203882014,-0.33909093068465,
-1.62691869420078));
#8962=CARTESIAN_POINT('Ctrl Pts',(-0.261368388670536,-0.317195968905306,
-1.62252828437015));
#8963=CARTESIAN_POINT('Ctrl Pts',(-0.311480544243686,-0.266264900654908,
-1.61365775139403));
#8964=CARTESIAN_POINT('Ctrl Pts',(-0.333298652394954,-0.237231147975234,
-1.60919314384089));
#8965=CARTESIAN_POINT('Ctrl Pts',(-0.373030350867485,-0.166543350814306,
-1.60050712143809));
#8966=CARTESIAN_POINT('Ctrl Pts',(-0.388626558458099,-0.123401821157026,
-1.59665523941937));
#8967=CARTESIAN_POINT('Ctrl Pts',(-0.397005914195118,-0.07938,-1.59456899932179));
#8968=CARTESIAN_POINT('Origin',(1.11022302462516E-16,-0.07938,-1.675));
#8969=CARTESIAN_POINT('Origin',(0.,-0.07938,0.));
#8970=CARTESIAN_POINT('',(0.846804978391753,-0.07938,-1.40825612658882));
#8971=CARTESIAN_POINT('Origin',(0.,-0.07938,0.));
#8972=CARTESIAN_POINT('Origin',(1.18440385848747,-0.07938,-1.18440385848747));
#8973=CARTESIAN_POINT('Origin',(1.18440385848747,0.,-1.18440385848747));
#8974=CARTESIAN_POINT('',(1.40825612658882,-0.07938,-0.846804978391753));
#8975=CARTESIAN_POINT('Ctrl Pts',(1.40825612658882,-0.0793800000000001,
-0.846804978391753));
#8976=CARTESIAN_POINT('Ctrl Pts',(1.40380622184538,-0.123401821157026,-0.854205272175555));
#8977=CARTESIAN_POINT('Ctrl Pts',(1.39550172959303,-0.166543350814306,-0.867957148219442));
#8978=CARTESIAN_POINT('Ctrl Pts',(1.3735491215176,-0.237231147975234,-0.902193646979983));
#8979=CARTESIAN_POINT('Ctrl Pts',(1.36127834356734,-0.266264900654908,-0.920778333482565));
#8980=CARTESIAN_POINT('Ctrl Pts',(1.33211611256184,-0.317195968905306,-0.962485392528369));
#8981=CARTESIAN_POINT('Ctrl Pts',(1.31521005565926,-0.33909093068465,-0.985600426557816));
#8982=CARTESIAN_POINT('Ctrl Pts',(1.27866649102984,-0.373586846396559,-1.03253285680459));
#8983=CARTESIAN_POINT('Ctrl Pts',(1.25722555095714,-0.388086240756494,-1.05871835910697));
#8984=CARTESIAN_POINT('Ctrl Pts',(1.2107812086231,-0.407068917407805,-1.11153475808518));
#8985=CARTESIAN_POINT('Ctrl Pts',(1.18575674747573,-0.411552957311693,-1.13814686046673));
#8986=CARTESIAN_POINT('Ctrl Pts',(1.13814686046673,-0.411552957311693,-1.18575674747573));
#8987=CARTESIAN_POINT('Ctrl Pts',(1.11153475808518,-0.407068917407805,-1.2107812086231));
#8988=CARTESIAN_POINT('Ctrl Pts',(1.05871835910697,-0.388086240756494,-1.25722555095714));
#8989=CARTESIAN_POINT('Ctrl Pts',(1.03253285680459,-0.373586846396559,-1.27866649102984));
#8990=CARTESIAN_POINT('Ctrl Pts',(0.985600426557816,-0.33909093068465,-1.31521005565926));
#8991=CARTESIAN_POINT('Ctrl Pts',(0.962485392528369,-0.317195968905306,
-1.33211611256184));
#8992=CARTESIAN_POINT('Ctrl Pts',(0.920778333482565,-0.266264900654909,
-1.36127834356734));
#8993=CARTESIAN_POINT('Ctrl Pts',(0.902193646979983,-0.237231147975234,
-1.3735491215176));
#8994=CARTESIAN_POINT('Ctrl Pts',(0.867957148219442,-0.166543350814306,
-1.39550172959303));
#8995=CARTESIAN_POINT('Ctrl Pts',(0.854205272175555,-0.123401821157026,
-1.40380622184538));
#8996=CARTESIAN_POINT('Ctrl Pts',(0.846804978391753,-0.0793800000000001,
-1.40825612658882));
#8997=CARTESIAN_POINT('Origin',(1.18440385848747,-0.07938,-1.18440385848747));
#8998=CARTESIAN_POINT('Origin',(0.,-0.27783,0.));
#8999=CARTESIAN_POINT('',(-1.643248,-0.47628,2.01239840340529E-16));
#9000=CARTESIAN_POINT('Origin',(0.,-0.47628,0.));
#9001=CARTESIAN_POINT('',(-1.643248,-0.27783,2.01239840340529E-16));
#9002=CARTESIAN_POINT('',(1.59456899932179,-0.07938,0.397005914195118));
#9003=CARTESIAN_POINT('Origin',(0.,-0.07938,0.));
#9004=CARTESIAN_POINT('',(1.59456899932179,-0.07938,-0.397005914195118));
#9005=CARTESIAN_POINT('Ctrl Pts',(1.59456899932179,-0.0793800000000001,
0.397005914195118));
#9006=CARTESIAN_POINT('Ctrl Pts',(1.59665523941937,-0.123401821157026,0.388626558458099));
#9007=CARTESIAN_POINT('Ctrl Pts',(1.60050712143809,-0.166543350814306,0.373030350867485));
#9008=CARTESIAN_POINT('Ctrl Pts',(1.60919314384089,-0.237231147975234,0.333298652394954));
#9009=CARTESIAN_POINT('Ctrl Pts',(1.61365775139403,-0.266264900654909,0.311480544243686));
#9010=CARTESIAN_POINT('Ctrl Pts',(1.62252828437015,-0.317195968905306,0.261368388670537));
#9011=CARTESIAN_POINT('Ctrl Pts',(1.62691869420078,-0.33909093068465,0.233069203882014));
#9012=CARTESIAN_POINT('Ctrl Pts',(1.63426473152765,-0.373586846396559,0.174042761838764));
#9013=CARTESIAN_POINT('Ctrl Pts',(1.63761964365402,-0.388086240756494,0.140365781471549));
#9014=CARTESIAN_POINT('Ctrl Pts',(1.64212536811722,-0.407068917407805,0.0701778381840612));
#9015=CARTESIAN_POINT('Ctrl Pts',(1.643248,-0.411552957311693,0.0336652739555916));
#9016=CARTESIAN_POINT('Ctrl Pts',(1.643248,-0.411552957311693,-0.0336652739555916));
#9017=CARTESIAN_POINT('Ctrl Pts',(1.64212536811722,-0.407068917407805,-0.0701778381840612));
#9018=CARTESIAN_POINT('Ctrl Pts',(1.63761964365402,-0.388086240756494,-0.140365781471549));
#9019=CARTESIAN_POINT('Ctrl Pts',(1.63426473152765,-0.373586846396559,-0.174042761838764));
#9020=CARTESIAN_POINT('Ctrl Pts',(1.62691869420078,-0.33909093068465,-0.233069203882014));
#9021=CARTESIAN_POINT('Ctrl Pts',(1.62252828437015,-0.317195968905306,-0.261368388670537));
#9022=CARTESIAN_POINT('Ctrl Pts',(1.61365775139403,-0.266264900654909,-0.311480544243686));
#9023=CARTESIAN_POINT('Ctrl Pts',(1.60919314384089,-0.237231147975234,-0.333298652394954));
#9024=CARTESIAN_POINT('Ctrl Pts',(1.60050712143809,-0.166543350814306,-0.373030350867485));
#9025=CARTESIAN_POINT('Ctrl Pts',(1.59665523941937,-0.123401821157026,-0.388626558458099));
#9026=CARTESIAN_POINT('Ctrl Pts',(1.59456899932179,-0.07938,-0.397005914195118));
#9027=CARTESIAN_POINT('Origin',(0.,-0.07938,0.));
#9028=CARTESIAN_POINT('Origin',(0.,-0.07938,0.));
#9029=CARTESIAN_POINT('Origin',(1.675,-0.07938,0.));
#9030=CARTESIAN_POINT('Origin',(1.675,0.,0.));
#9031=CARTESIAN_POINT('Origin',(1.675,-0.07938,0.));
#9032=CARTESIAN_POINT('Origin',(0.,-0.47628,0.));
#9033=CARTESIAN_POINT('Origin',(0.,-0.07938,0.));
#9345=UNCERTAINTY_MEASURE_WITH_UNIT(LENGTH_MEASURE(0.001),#9392,
'DISTANCE_ACCURACY_VALUE',
'Maximum model space distance between geometric entities at asserted c
onnectivities');
#9354=UNCERTAINTY_MEASURE_WITH_UNIT(LENGTH_MEASURE(0.001),#9392,
'DISTANCE_ACCURACY_VALUE',
'Maximum model space distance between geometric entities at asserted c
onnectivities');
#9382=(
GEOMETRIC_REPRESENTATION_CONTEXT(3)
GLOBAL_UNCERTAINTY_ASSIGNED_CONTEXT((#9345))
GLOBAL_UNIT_ASSIGNED_CONTEXT((#9392,#9394,#9395))
REPRESENTATION_CONTEXT('','3D')
);
#9391=(
GEOMETRIC_REPRESENTATION_CONTEXT(3)
GLOBAL_UNCERTAINTY_ASSIGNED_CONTEXT((#9354))
GLOBAL_UNIT_ASSIGNED_CONTEXT((#9392,#9394,#9395))
REPRESENTATION_CONTEXT('','3D')
);
#9392=(
LENGTH_UNIT()
NAMED_UNIT(*)
SI_UNIT(.CENTI.,.METRE.)
);
#9394=(
NAMED_UNIT(*)
PLANE_ANGLE_UNIT()
SI_UNIT($,.RADIAN.)
);
#9395=(
NAMED_UNIT(*)
SI_UNIT($,.STERADIAN.)
SOLID_ANGLE_UNIT()
);
#9423=SHAPE_DEFINITION_REPRESENTATION(#9484,#9547);
#9484=PRODUCT_DEFINITION_SHAPE('',$,#9584);
#9547=SHAPE_REPRESENTATION('',(#5740),#9382);
#9556=PRODUCT_DEFINITION_CONTEXT('part definition',#9666,'design');
#9584=PRODUCT_DEFINITION('Cage','Cage',#9620,#9556);
#9620=PRODUCT_DEFINITION_FORMATION('',$,#9695);
#9666=APPLICATION_CONTEXT(
'Core Data for Automotive Mechanical Design Process');
#9667=PRODUCT_CONTEXT('part definition',#9666,'mechanical');
#9695=PRODUCT('Cage','Cage','Cage',(#9667));
#9753=COLOUR_RGB('Grey',0.48,0.52,0.57);
#9754=FILL_AREA_STYLE_COLOUR('',#9753);
#9755=FILL_AREA_STYLE('',(#9754));
#9756=SURFACE_STYLE_FILL_AREA(#9755);
#9757=SURFACE_SIDE_STYLE('',(#9756));
#9758=SURFACE_STYLE_USAGE(.BOTH.,#9757);
#9759=PRESENTATION_STYLE_ASSIGNMENT((#9758));
ENDSEC;
END-ISO-10303-21;
